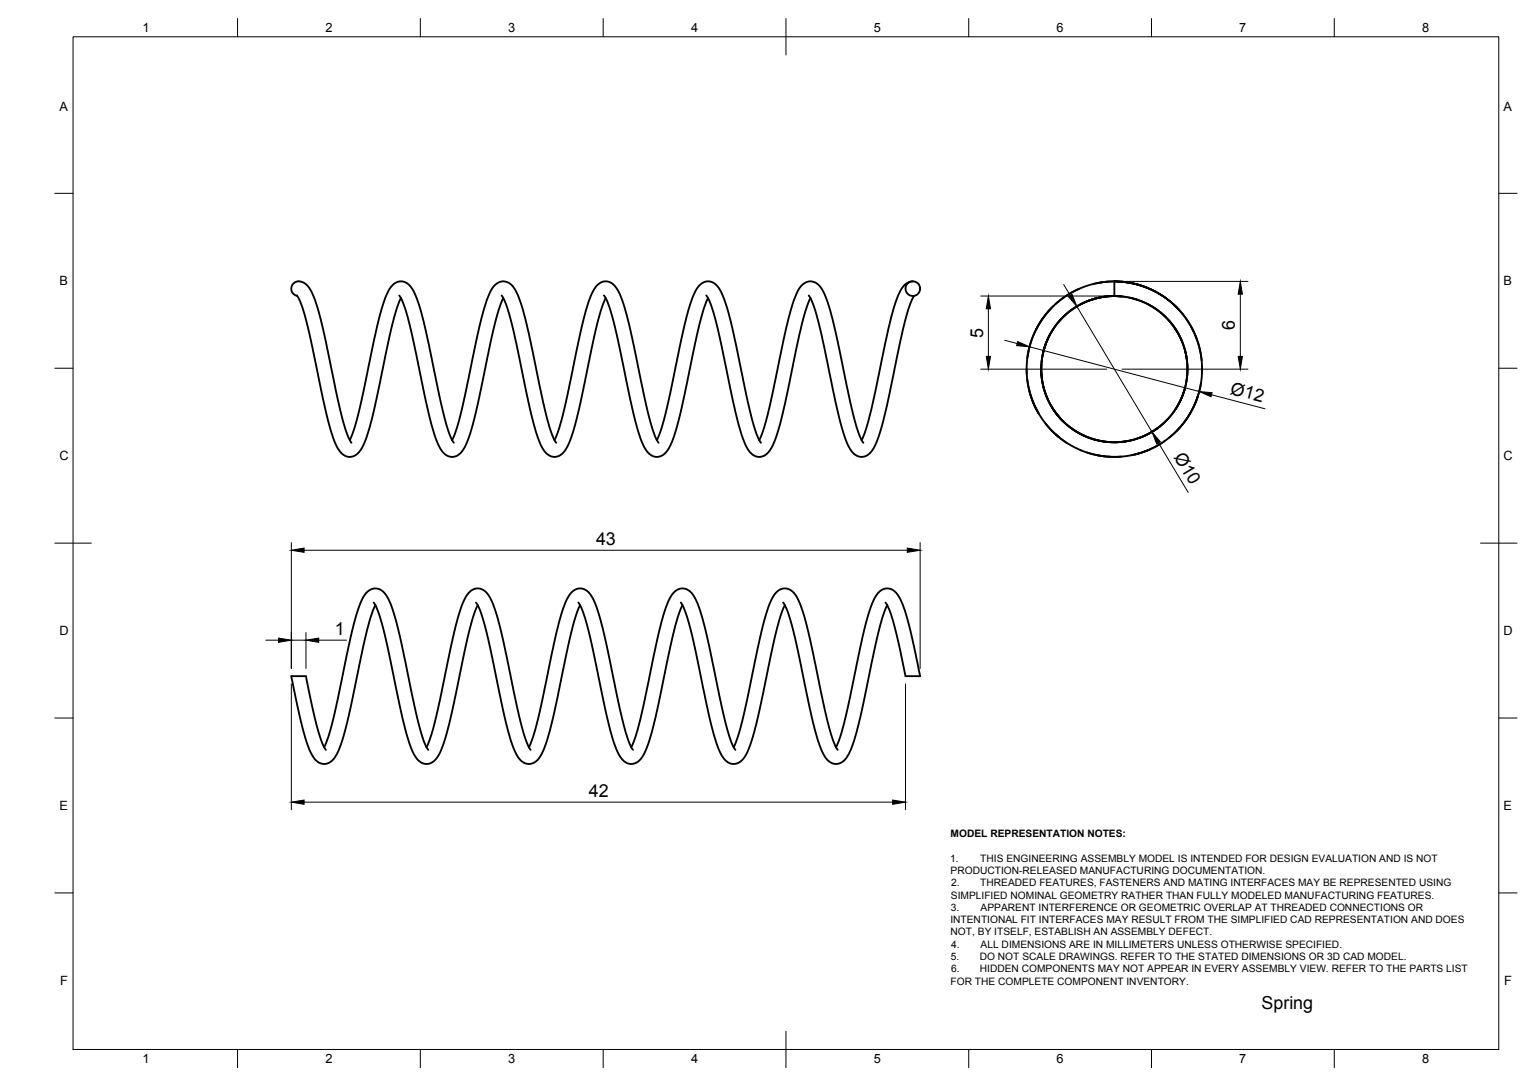
ISO-10303-21;
HEADER;
/* Generated by software containing ST-Developer
 * from STEP Tools, Inc. (www.steptools.com) 
 */

FILE_DESCRIPTION(
/* description */ (''),
/* implementation_level */ '2;1');

FILE_NAME(
/* name */ 'Spring.step',
/* time_stamp */ '2026-10-06T13:05:37-07:00',
/* author */ (''),
/* organization */ (''),
/* preprocessor_version */ 'ST-DEVELOPER v20.2',
/* originating_system */ 'Autodesk Translation Framework v15.15.0.0',
/* authorisation */ '');

FILE_SCHEMA (('AUTOMOTIVE_DESIGN { 1 0 10303 214 3 1 1 }'));
ENDSEC;

DATA;
#10=MECHANICAL_DESIGN_GEOMETRIC_PRESENTATION_REPRESENTATION('',(#145),#28055);
#96=B_SPLINE_SURFACE_WITH_KNOTS('',3,3,((#25876,#25877,#25878,#25879,#25880,
#25881,#25882,#25883,#25884,#25885,#25886,#25887,#25888,#25889,#25890,#25891,
#25892,#25893,#25894,#25895,#25896,#25897,#25898,#25899,#25900,#25901,#25902,
#25903,#25904,#25905,#25906,#25907,#25908,#25909,#25910,#25911,#25912,#25913,
#25914,#25915,#25916,#25917,#25918,#25919,#25920,#25921,#25922,#25923,#25924,
#25925,#25926,#25927,#25928,#25929,#25930,#25931,#25932,#25933,#25934,#25935,
#25936,#25937,#25938,#25939,#25940,#25941,#25942,#25943,#25944,#25945,#25946,
#25947,#25948,#25949,#25950,#25951,#25952,#25953,#25954),(#25955,#25956,
#25957,#25958,#25959,#25960,#25961,#25962,#25963,#25964,#25965,#25966,#25967,
#25968,#25969,#25970,#25971,#25972,#25973,#25974,#25975,#25976,#25977,#25978,
#25979,#25980,#25981,#25982,#25983,#25984,#25985,#25986,#25987,#25988,#25989,
#25990,#25991,#25992,#25993,#25994,#25995,#25996,#25997,#25998,#25999,#26000,
#26001,#26002,#26003,#26004,#26005,#26006,#26007,#26008,#26009,#26010,#26011,
#26012,#26013,#26014,#26015,#26016,#26017,#26018,#26019,#26020,#26021,#26022,
#26023,#26024,#26025,#26026,#26027,#26028,#26029,#26030,#26031,#26032,#26033),
(#26034,#26035,#26036,#26037,#26038,#26039,#26040,#26041,#26042,#26043,
#26044,#26045,#26046,#26047,#26048,#26049,#26050,#26051,#26052,#26053,#26054,
#26055,#26056,#26057,#26058,#26059,#26060,#26061,#26062,#26063,#26064,#26065,
#26066,#26067,#26068,#26069,#26070,#26071,#26072,#26073,#26074,#26075,#26076,
#26077,#26078,#26079,#26080,#26081,#26082,#26083,#26084,#26085,#26086,#26087,
#26088,#26089,#26090,#26091,#26092,#26093,#26094,#26095,#26096,#26097,#26098,
#26099,#26100,#26101,#26102,#26103,#26104,#26105,#26106,#26107,#26108,#26109,
#26110,#26111,#26112),(#26113,#26114,#26115,#26116,#26117,#26118,#26119,
#26120,#26121,#26122,#26123,#26124,#26125,#26126,#26127,#26128,#26129,#26130,
#26131,#26132,#26133,#26134,#26135,#26136,#26137,#26138,#26139,#26140,#26141,
#26142,#26143,#26144,#26145,#26146,#26147,#26148,#26149,#26150,#26151,#26152,
#26153,#26154,#26155,#26156,#26157,#26158,#26159,#26160,#26161,#26162,#26163,
#26164,#26165,#26166,#26167,#26168,#26169,#26170,#26171,#26172,#26173,#26174,
#26175,#26176,#26177,#26178,#26179,#26180,#26181,#26182,#26183,#26184,#26185,
#26186,#26187,#26188,#26189,#26190,#26191),(#26192,#26193,#26194,#26195,
#26196,#26197,#26198,#26199,#26200,#26201,#26202,#26203,#26204,#26205,#26206,
#26207,#26208,#26209,#26210,#26211,#26212,#26213,#26214,#26215,#26216,#26217,
#26218,#26219,#26220,#26221,#26222,#26223,#26224,#26225,#26226,#26227,#26228,
#26229,#26230,#26231,#26232,#26233,#26234,#26235,#26236,#26237,#26238,#26239,
#26240,#26241,#26242,#26243,#26244,#26245,#26246,#26247,#26248,#26249,#26250,
#26251,#26252,#26253,#26254,#26255,#26256,#26257,#26258,#26259,#26260,#26261,
#26262,#26263,#26264,#26265,#26266,#26267,#26268,#26269,#26270),(#26271,
#26272,#26273,#26274,#26275,#26276,#26277,#26278,#26279,#26280,#26281,#26282,
#26283,#26284,#26285,#26286,#26287,#26288,#26289,#26290,#26291,#26292,#26293,
#26294,#26295,#26296,#26297,#26298,#26299,#26300,#26301,#26302,#26303,#26304,
#26305,#26306,#26307,#26308,#26309,#26310,#26311,#26312,#26313,#26314,#26315,
#26316,#26317,#26318,#26319,#26320,#26321,#26322,#26323,#26324,#26325,#26326,
#26327,#26328,#26329,#26330,#26331,#26332,#26333,#26334,#26335,#26336,#26337,
#26338,#26339,#26340,#26341,#26342,#26343,#26344,#26345,#26346,#26347,#26348,
#26349),(#26350,#26351,#26352,#26353,#26354,#26355,#26356,#26357,#26358,
#26359,#26360,#26361,#26362,#26363,#26364,#26365,#26366,#26367,#26368,#26369,
#26370,#26371,#26372,#26373,#26374,#26375,#26376,#26377,#26378,#26379,#26380,
#26381,#26382,#26383,#26384,#26385,#26386,#26387,#26388,#26389,#26390,#26391,
#26392,#26393,#26394,#26395,#26396,#26397,#26398,#26399,#26400,#26401,#26402,
#26403,#26404,#26405,#26406,#26407,#26408,#26409,#26410,#26411,#26412,#26413,
#26414,#26415,#26416,#26417,#26418,#26419,#26420,#26421,#26422,#26423,#26424,
#26425,#26426,#26427,#26428),(#26429,#26430,#26431,#26432,#26433,#26434,
#26435,#26436,#26437,#26438,#26439,#26440,#26441,#26442,#26443,#26444,#26445,
#26446,#26447,#26448,#26449,#26450,#26451,#26452,#26453,#26454,#26455,#26456,
#26457,#26458,#26459,#26460,#26461,#26462,#26463,#26464,#26465,#26466,#26467,
#26468,#26469,#26470,#26471,#26472,#26473,#26474,#26475,#26476,#26477,#26478,
#26479,#26480,#26481,#26482,#26483,#26484,#26485,#26486,#26487,#26488,#26489,
#26490,#26491,#26492,#26493,#26494,#26495,#26496,#26497,#26498,#26499,#26500,
#26501,#26502,#26503,#26504,#26505,#26506,#26507),(#26508,#26509,#26510,
#26511,#26512,#26513,#26514,#26515,#26516,#26517,#26518,#26519,#26520,#26521,
#26522,#26523,#26524,#26525,#26526,#26527,#26528,#26529,#26530,#26531,#26532,
#26533,#26534,#26535,#26536,#26537,#26538,#26539,#26540,#26541,#26542,#26543,
#26544,#26545,#26546,#26547,#26548,#26549,#26550,#26551,#26552,#26553,#26554,
#26555,#26556,#26557,#26558,#26559,#26560,#26561,#26562,#26563,#26564,#26565,
#26566,#26567,#26568,#26569,#26570,#26571,#26572,#26573,#26574,#26575,#26576,
#26577,#26578,#26579,#26580,#26581,#26582,#26583,#26584,#26585,#26586),
(#26587,#26588,#26589,#26590,#26591,#26592,#26593,#26594,#26595,#26596,
#26597,#26598,#26599,#26600,#26601,#26602,#26603,#26604,#26605,#26606,#26607,
#26608,#26609,#26610,#26611,#26612,#26613,#26614,#26615,#26616,#26617,#26618,
#26619,#26620,#26621,#26622,#26623,#26624,#26625,#26626,#26627,#26628,#26629,
#26630,#26631,#26632,#26633,#26634,#26635,#26636,#26637,#26638,#26639,#26640,
#26641,#26642,#26643,#26644,#26645,#26646,#26647,#26648,#26649,#26650,#26651,
#26652,#26653,#26654,#26655,#26656,#26657,#26658,#26659,#26660,#26661,#26662,
#26663,#26664,#26665),(#26666,#26667,#26668,#26669,#26670,#26671,#26672,
#26673,#26674,#26675,#26676,#26677,#26678,#26679,#26680,#26681,#26682,#26683,
#26684,#26685,#26686,#26687,#26688,#26689,#26690,#26691,#26692,#26693,#26694,
#26695,#26696,#26697,#26698,#26699,#26700,#26701,#26702,#26703,#26704,#26705,
#26706,#26707,#26708,#26709,#26710,#26711,#26712,#26713,#26714,#26715,#26716,
#26717,#26718,#26719,#26720,#26721,#26722,#26723,#26724,#26725,#26726,#26727,
#26728,#26729,#26730,#26731,#26732,#26733,#26734,#26735,#26736,#26737,#26738,
#26739,#26740,#26741,#26742,#26743,#26744),(#26745,#26746,#26747,#26748,
#26749,#26750,#26751,#26752,#26753,#26754,#26755,#26756,#26757,#26758,#26759,
#26760,#26761,#26762,#26763,#26764,#26765,#26766,#26767,#26768,#26769,#26770,
#26771,#26772,#26773,#26774,#26775,#26776,#26777,#26778,#26779,#26780,#26781,
#26782,#26783,#26784,#26785,#26786,#26787,#26788,#26789,#26790,#26791,#26792,
#26793,#26794,#26795,#26796,#26797,#26798,#26799,#26800,#26801,#26802,#26803,
#26804,#26805,#26806,#26807,#26808,#26809,#26810,#26811,#26812,#26813,#26814,
#26815,#26816,#26817,#26818,#26819,#26820,#26821,#26822,#26823)),
 .UNSPECIFIED.,.T.,.F.,.F.,(4,1,1,1,2,1,1,1,4),(4,1,1,1,1,1,1,1,1,1,1,1,
1,1,1,1,1,1,1,1,1,1,1,1,1,1,1,1,1,1,1,1,1,1,1,1,1,1,1,1,1,1,1,1,1,1,1,1,
1,1,1,1,1,1,1,1,1,1,1,1,1,1,1,1,1,1,1,1,1,1,1,1,1,1,1,1,4),(-6.28318530717958,
-5.83438635666675,-4.9367884556411,-4.03919055461544,-3.14159265358979,
-2.24399475256414,-1.34639685153848,-0.448798950512828,0.),(0.,0.496040945303652,
0.992081890607303,1.48812283591095,1.98416378121461,2.48020472651826,2.97624567182191,
3.47228661712556,3.96832756242921,4.46436850773286,4.96040945303652,5.45645039834017,
5.95249134364382,6.44853228894747,6.94457323425112,7.44061417955477,7.93665512485842,
8.43269607016208,8.92873701546573,9.42477796076938,9.92081890607303,10.4168598513767,
10.9129007966803,11.408941741984,11.9049826872876,12.4010236325913,12.8970645778949,
13.3931055231986,13.8891464685022,14.3851874138059,14.8812283591095,15.3772693044132,
15.8733102497168,16.3693511950205,16.8653921403242,17.3614330856278,17.8574740309315,
18.3535149762351,18.8495559215388,19.3455968668424,19.8416378121461,20.3376787574497,
20.8337197027534,21.329760648057,21.8258015933607,22.3218425386643,22.817883483968,
23.3139244292716,23.8099653745753,24.3060063198789,24.8020472651826,25.2980882104862,
25.7941291557899,26.2901701010935,26.7862110463972,27.2822519917008,27.7782929370045,
28.2743338823081,28.7703748276118,29.2664157729154,29.7624567182191,30.2584976635227,
30.7545386088264,31.25057955413,31.7466204994337,32.2426614447374,32.738702390041,
33.2347433353447,33.7307842806483,34.226825225952,34.7228661712556,35.2189071165593,
35.7149480618629,36.2109890071666,36.7070299524702,37.2030708977739,37.6991118430775),
 .UNSPECIFIED.);
#97=B_SPLINE_SURFACE_WITH_KNOTS('',3,3,((#27026,#27027,#27028,#27029,#27030,
#27031,#27032,#27033,#27034,#27035,#27036,#27037,#27038,#27039,#27040,#27041,
#27042,#27043,#27044,#27045,#27046,#27047,#27048,#27049,#27050,#27051,#27052,
#27053,#27054,#27055,#27056,#27057,#27058,#27059,#27060,#27061,#27062,#27063,
#27064,#27065,#27066,#27067,#27068,#27069,#27070,#27071,#27072,#27073,#27074,
#27075,#27076,#27077,#27078,#27079,#27080,#27081,#27082,#27083,#27084,#27085,
#27086,#27087,#27088,#27089,#27090,#27091,#27092,#27093,#27094,#27095,#27096,
#27097,#27098,#27099,#27100,#27101,#27102,#27103,#27104),(#27105,#27106,
#27107,#27108,#27109,#27110,#27111,#27112,#27113,#27114,#27115,#27116,#27117,
#27118,#27119,#27120,#27121,#27122,#27123,#27124,#27125,#27126,#27127,#27128,
#27129,#27130,#27131,#27132,#27133,#27134,#27135,#27136,#27137,#27138,#27139,
#27140,#27141,#27142,#27143,#27144,#27145,#27146,#27147,#27148,#27149,#27150,
#27151,#27152,#27153,#27154,#27155,#27156,#27157,#27158,#27159,#27160,#27161,
#27162,#27163,#27164,#27165,#27166,#27167,#27168,#27169,#27170,#27171,#27172,
#27173,#27174,#27175,#27176,#27177,#27178,#27179,#27180,#27181,#27182,#27183),
(#27184,#27185,#27186,#27187,#27188,#27189,#27190,#27191,#27192,#27193,
#27194,#27195,#27196,#27197,#27198,#27199,#27200,#27201,#27202,#27203,#27204,
#27205,#27206,#27207,#27208,#27209,#27210,#27211,#27212,#27213,#27214,#27215,
#27216,#27217,#27218,#27219,#27220,#27221,#27222,#27223,#27224,#27225,#27226,
#27227,#27228,#27229,#27230,#27231,#27232,#27233,#27234,#27235,#27236,#27237,
#27238,#27239,#27240,#27241,#27242,#27243,#27244,#27245,#27246,#27247,#27248,
#27249,#27250,#27251,#27252,#27253,#27254,#27255,#27256,#27257,#27258,#27259,
#27260,#27261,#27262),(#27263,#27264,#27265,#27266,#27267,#27268,#27269,
#27270,#27271,#27272,#27273,#27274,#27275,#27276,#27277,#27278,#27279,#27280,
#27281,#27282,#27283,#27284,#27285,#27286,#27287,#27288,#27289,#27290,#27291,
#27292,#27293,#27294,#27295,#27296,#27297,#27298,#27299,#27300,#27301,#27302,
#27303,#27304,#27305,#27306,#27307,#27308,#27309,#27310,#27311,#27312,#27313,
#27314,#27315,#27316,#27317,#27318,#27319,#27320,#27321,#27322,#27323,#27324,
#27325,#27326,#27327,#27328,#27329,#27330,#27331,#27332,#27333,#27334,#27335,
#27336,#27337,#27338,#27339,#27340,#27341),(#27342,#27343,#27344,#27345,
#27346,#27347,#27348,#27349,#27350,#27351,#27352,#27353,#27354,#27355,#27356,
#27357,#27358,#27359,#27360,#27361,#27362,#27363,#27364,#27365,#27366,#27367,
#27368,#27369,#27370,#27371,#27372,#27373,#27374,#27375,#27376,#27377,#27378,
#27379,#27380,#27381,#27382,#27383,#27384,#27385,#27386,#27387,#27388,#27389,
#27390,#27391,#27392,#27393,#27394,#27395,#27396,#27397,#27398,#27399,#27400,
#27401,#27402,#27403,#27404,#27405,#27406,#27407,#27408,#27409,#27410,#27411,
#27412,#27413,#27414,#27415,#27416,#27417,#27418,#27419,#27420),(#27421,
#27422,#27423,#27424,#27425,#27426,#27427,#27428,#27429,#27430,#27431,#27432,
#27433,#27434,#27435,#27436,#27437,#27438,#27439,#27440,#27441,#27442,#27443,
#27444,#27445,#27446,#27447,#27448,#27449,#27450,#27451,#27452,#27453,#27454,
#27455,#27456,#27457,#27458,#27459,#27460,#27461,#27462,#27463,#27464,#27465,
#27466,#27467,#27468,#27469,#27470,#27471,#27472,#27473,#27474,#27475,#27476,
#27477,#27478,#27479,#27480,#27481,#27482,#27483,#27484,#27485,#27486,#27487,
#27488,#27489,#27490,#27491,#27492,#27493,#27494,#27495,#27496,#27497,#27498,
#27499),(#27500,#27501,#27502,#27503,#27504,#27505,#27506,#27507,#27508,
#27509,#27510,#27511,#27512,#27513,#27514,#27515,#27516,#27517,#27518,#27519,
#27520,#27521,#27522,#27523,#27524,#27525,#27526,#27527,#27528,#27529,#27530,
#27531,#27532,#27533,#27534,#27535,#27536,#27537,#27538,#27539,#27540,#27541,
#27542,#27543,#27544,#27545,#27546,#27547,#27548,#27549,#27550,#27551,#27552,
#27553,#27554,#27555,#27556,#27557,#27558,#27559,#27560,#27561,#27562,#27563,
#27564,#27565,#27566,#27567,#27568,#27569,#27570,#27571,#27572,#27573,#27574,
#27575,#27576,#27577,#27578),(#27579,#27580,#27581,#27582,#27583,#27584,
#27585,#27586,#27587,#27588,#27589,#27590,#27591,#27592,#27593,#27594,#27595,
#27596,#27597,#27598,#27599,#27600,#27601,#27602,#27603,#27604,#27605,#27606,
#27607,#27608,#27609,#27610,#27611,#27612,#27613,#27614,#27615,#27616,#27617,
#27618,#27619,#27620,#27621,#27622,#27623,#27624,#27625,#27626,#27627,#27628,
#27629,#27630,#27631,#27632,#27633,#27634,#27635,#27636,#27637,#27638,#27639,
#27640,#27641,#27642,#27643,#27644,#27645,#27646,#27647,#27648,#27649,#27650,
#27651,#27652,#27653,#27654,#27655,#27656,#27657),(#27658,#27659,#27660,
#27661,#27662,#27663,#27664,#27665,#27666,#27667,#27668,#27669,#27670,#27671,
#27672,#27673,#27674,#27675,#27676,#27677,#27678,#27679,#27680,#27681,#27682,
#27683,#27684,#27685,#27686,#27687,#27688,#27689,#27690,#27691,#27692,#27693,
#27694,#27695,#27696,#27697,#27698,#27699,#27700,#27701,#27702,#27703,#27704,
#27705,#27706,#27707,#27708,#27709,#27710,#27711,#27712,#27713,#27714,#27715,
#27716,#27717,#27718,#27719,#27720,#27721,#27722,#27723,#27724,#27725,#27726,
#27727,#27728,#27729,#27730,#27731,#27732,#27733,#27734,#27735,#27736),
(#27737,#27738,#27739,#27740,#27741,#27742,#27743,#27744,#27745,#27746,
#27747,#27748,#27749,#27750,#27751,#27752,#27753,#27754,#27755,#27756,#27757,
#27758,#27759,#27760,#27761,#27762,#27763,#27764,#27765,#27766,#27767,#27768,
#27769,#27770,#27771,#27772,#27773,#27774,#27775,#27776,#27777,#27778,#27779,
#27780,#27781,#27782,#27783,#27784,#27785,#27786,#27787,#27788,#27789,#27790,
#27791,#27792,#27793,#27794,#27795,#27796,#27797,#27798,#27799,#27800,#27801,
#27802,#27803,#27804,#27805,#27806,#27807,#27808,#27809,#27810,#27811,#27812,
#27813,#27814,#27815),(#27816,#27817,#27818,#27819,#27820,#27821,#27822,
#27823,#27824,#27825,#27826,#27827,#27828,#27829,#27830,#27831,#27832,#27833,
#27834,#27835,#27836,#27837,#27838,#27839,#27840,#27841,#27842,#27843,#27844,
#27845,#27846,#27847,#27848,#27849,#27850,#27851,#27852,#27853,#27854,#27855,
#27856,#27857,#27858,#27859,#27860,#27861,#27862,#27863,#27864,#27865,#27866,
#27867,#27868,#27869,#27870,#27871,#27872,#27873,#27874,#27875,#27876,#27877,
#27878,#27879,#27880,#27881,#27882,#27883,#27884,#27885,#27886,#27887,#27888,
#27889,#27890,#27891,#27892,#27893,#27894),(#27895,#27896,#27897,#27898,
#27899,#27900,#27901,#27902,#27903,#27904,#27905,#27906,#27907,#27908,#27909,
#27910,#27911,#27912,#27913,#27914,#27915,#27916,#27917,#27918,#27919,#27920,
#27921,#27922,#27923,#27924,#27925,#27926,#27927,#27928,#27929,#27930,#27931,
#27932,#27933,#27934,#27935,#27936,#27937,#27938,#27939,#27940,#27941,#27942,
#27943,#27944,#27945,#27946,#27947,#27948,#27949,#27950,#27951,#27952,#27953,
#27954,#27955,#27956,#27957,#27958,#27959,#27960,#27961,#27962,#27963,#27964,
#27965,#27966,#27967,#27968,#27969,#27970,#27971,#27972,#27973)),
 .UNSPECIFIED.,.T.,.F.,.F.,(4,1,1,1,2,1,1,1,4),(4,1,1,1,1,1,1,1,1,1,1,1,
1,1,1,1,1,1,1,1,1,1,1,1,1,1,1,1,1,1,1,1,1,1,1,1,1,1,1,1,1,1,1,1,1,1,1,1,
1,1,1,1,1,1,1,1,1,1,1,1,1,1,1,1,1,1,1,1,1,1,1,1,1,1,1,1,4),(6.28318530717958,
6.73198425769241,7.62958215871806,8.52718005974372,9.42477796076937,10.322375861795,
11.2199737628207,12.1175716638463,12.5663706143592),(0.,0.496040945303652,
0.992081890607303,1.48812283591095,1.98416378121461,2.48020472651826,2.97624567182191,
3.47228661712556,3.96832756242921,4.46436850773286,4.96040945303652,5.45645039834017,
5.95249134364382,6.44853228894747,6.94457323425112,7.44061417955477,7.93665512485842,
8.43269607016208,8.92873701546573,9.42477796076938,9.92081890607303,10.4168598513767,
10.9129007966803,11.408941741984,11.9049826872876,12.4010236325913,12.8970645778949,
13.3931055231986,13.8891464685022,14.3851874138059,14.8812283591095,15.3772693044132,
15.8733102497168,16.3693511950205,16.8653921403242,17.3614330856278,17.8574740309315,
18.3535149762351,18.8495559215388,19.3455968668424,19.8416378121461,20.3376787574497,
20.8337197027534,21.329760648057,21.8258015933607,22.3218425386643,22.817883483968,
23.3139244292716,23.8099653745753,24.3060063198789,24.8020472651826,25.2980882104862,
25.7941291557899,26.2901701010935,26.7862110463972,27.2822519917008,27.7782929370045,
28.2743338823081,28.7703748276118,29.2664157729154,29.7624567182191,30.2584976635227,
30.7545386088264,31.25057955413,31.7466204994337,32.2426614447374,32.738702390041,
33.2347433353447,33.7307842806483,34.226825225952,34.7228661712556,35.2189071165593,
35.7149480618629,36.2109890071666,36.7070299524702,37.2030708977739,37.6991118430775),
 .UNSPECIFIED.);
#125=SHAPE_REPRESENTATION_RELATIONSHIP('SRR','None',#28102,#135);
#135=ADVANCED_BREP_SHAPE_REPRESENTATION('',(#154),#28054);
#145=STYLED_ITEM('',(#28152),#154);
#154=MANIFOLD_SOLID_BREP('Body1',#3688);
#254=PLANE('',#4102);
#255=PLANE('',#4103);
#581=FACE_OUTER_BOUND('',#817,.T.);
#582=FACE_OUTER_BOUND('',#818,.T.);
#583=FACE_OUTER_BOUND('',#819,.T.);
#584=FACE_OUTER_BOUND('',#820,.T.);
#817=EDGE_LOOP('',(#3382,#3383,#3384,#3385));
#818=EDGE_LOOP('',(#3386,#3387,#3388,#3389));
#819=EDGE_LOOP('',(#3390,#3391));
#820=EDGE_LOOP('',(#3392,#3393));
#1388=B_SPLINE_CURVE_WITH_KNOTS('',3,(#26826,#26827,#26828,#26829,#26830,
#26831,#26832,#26833,#26834,#26835,#26836,#26837,#26838,#26839,#26840,#26841,
#26842,#26843,#26844,#26845,#26846,#26847,#26848,#26849,#26850,#26851,#26852,
#26853,#26854,#26855,#26856,#26857,#26858,#26859,#26860,#26861,#26862,#26863,
#26864,#26865,#26866,#26867,#26868,#26869,#26870,#26871,#26872,#26873,#26874,
#26875,#26876,#26877,#26878,#26879,#26880,#26881,#26882,#26883,#26884,#26885,
#26886,#26887,#26888,#26889,#26890,#26891,#26892,#26893,#26894,#26895,#26896,
#26897,#26898,#26899,#26900,#26901,#26902,#26903,#26904),.UNSPECIFIED.,
 .F.,.F.,(4,1,1,1,1,1,1,1,1,1,1,1,1,1,1,1,1,1,1,1,1,1,1,1,1,1,1,1,1,1,1,
1,1,1,1,1,1,1,1,1,1,1,1,1,1,1,1,1,1,1,1,1,1,1,1,1,1,1,1,1,1,1,1,1,1,1,1,
1,1,1,1,1,1,1,1,1,4),(-37.6991118430775,-37.2030708977739,-36.7070299524702,
-36.2109890071666,-35.7149480618629,-35.2189071165593,-34.7228661712556,
-34.226825225952,-33.7307842806483,-33.2347433353447,-32.738702390041,-32.2426614447374,
-31.7466204994337,-31.25057955413,-30.7545386088264,-30.2584976635227,-29.7624567182191,
-29.2664157729154,-28.7703748276118,-28.2743338823081,-27.7782929370045,
-27.2822519917008,-26.7862110463972,-26.2901701010935,-25.7941291557899,
-25.2980882104862,-24.8020472651826,-24.3060063198789,-23.8099653745753,
-23.3139244292716,-22.817883483968,-22.3218425386643,-21.8258015933607,
-21.329760648057,-20.8337197027534,-20.3376787574497,-19.8416378121461,
-19.3455968668424,-18.8495559215388,-18.3535149762351,-17.8574740309315,
-17.3614330856278,-16.8653921403242,-16.3693511950205,-15.8733102497168,
-15.3772693044132,-14.8812283591095,-14.3851874138059,-13.8891464685022,
-13.3931055231986,-12.8970645778949,-12.4010236325913,-11.9049826872876,
-11.408941741984,-10.9129007966803,-10.4168598513767,-9.92081890607303,
-9.42477796076938,-8.92873701546573,-8.43269607016208,-7.93665512485842,
-7.44061417955477,-6.94457323425112,-6.44853228894747,-5.95249134364382,
-5.45645039834017,-4.96040945303652,-4.46436850773286,-3.96832756242921,
-3.47228661712556,-2.97624567182191,-2.48020472651826,-1.98416378121461,
-1.48812283591095,-0.992081890607303,-0.496040945303652,0.),
 .UNSPECIFIED.);
#1389=B_SPLINE_CURVE_WITH_KNOTS('',3,(#26906,#26907,#26908,#26909,#26910,
#26911,#26912,#26913,#26914,#26915,#26916,#26917,#26918,#26919,#26920,#26921,
#26922,#26923,#26924,#26925),.UNSPECIFIED.,.F.,.F.,(4,2,2,2,2,2,2,2,2,4),
(-0.183449247657807,-0.181303576912795,-0.161079000210457,-0.142089796258872,
-0.119840622322675,-0.0936636492746921,-0.0676644266740556,-0.0408453735972391,
-0.019825886307719,-2.33571946147655E-5),.UNSPECIFIED.);
#1390=B_SPLINE_CURVE_WITH_KNOTS('',3,(#26927,#26928,#26929,#26930,#26931,
#26932,#26933,#26934,#26935,#26936,#26937,#26938,#26939,#26940,#26941,#26942,
#26943,#26944,#26945,#26946,#26947,#26948,#26949,#26950,#26951,#26952,#26953,
#26954,#26955,#26956,#26957,#26958,#26959,#26960,#26961,#26962,#26963,#26964,
#26965,#26966,#26967,#26968,#26969,#26970,#26971,#26972,#26973,#26974,#26975,
#26976,#26977,#26978,#26979,#26980,#26981,#26982,#26983,#26984,#26985,#26986,
#26987,#26988,#26989,#26990,#26991,#26992,#26993,#26994,#26995,#26996,#26997,
#26998,#26999,#27000,#27001,#27002,#27003,#27004,#27005),.UNSPECIFIED.,
 .F.,.F.,(4,1,1,1,1,1,1,1,1,1,1,1,1,1,1,1,1,1,1,1,1,1,1,1,1,1,1,1,1,1,1,
1,1,1,1,1,1,1,1,1,1,1,1,1,1,1,1,1,1,1,1,1,1,1,1,1,1,1,1,1,1,1,1,1,1,1,1,
1,1,1,1,1,1,1,1,1,4),(0.,0.496040945303652,0.992081890607303,1.48812283591095,
1.98416378121461,2.48020472651826,2.97624567182191,3.47228661712556,3.96832756242921,
4.46436850773286,4.96040945303652,5.45645039834017,5.95249134364382,6.44853228894747,
6.94457323425112,7.44061417955477,7.93665512485842,8.43269607016208,8.92873701546573,
9.42477796076938,9.92081890607303,10.4168598513767,10.9129007966803,11.408941741984,
11.9049826872876,12.4010236325913,12.8970645778949,13.3931055231986,13.8891464685022,
14.3851874138059,14.8812283591095,15.3772693044132,15.8733102497168,16.3693511950205,
16.8653921403242,17.3614330856278,17.8574740309315,18.3535149762351,18.8495559215388,
19.3455968668424,19.8416378121461,20.3376787574497,20.8337197027534,21.329760648057,
21.8258015933607,22.3218425386643,22.817883483968,23.3139244292716,23.8099653745753,
24.3060063198789,24.8020472651826,25.2980882104862,25.7941291557899,26.2901701010935,
26.7862110463972,27.2822519917008,27.7782929370045,28.2743338823081,28.7703748276118,
29.2664157729154,29.7624567182191,30.2584976635227,30.7545386088264,31.25057955413,
31.7466204994337,32.2426614447374,32.738702390041,33.2347433353447,33.7307842806483,
34.226825225952,34.7228661712556,35.2189071165593,35.7149480618629,36.2109890071666,
36.7070299524702,37.2030708977739,37.6991118430775),.UNSPECIFIED.);
#1391=B_SPLINE_CURVE_WITH_KNOTS('',3,(#27006,#27007,#27008,#27009,#27010,
#27011,#27012,#27013,#27014,#27015,#27016,#27017,#27018,#27019,#27020,#27021,
#27022,#27023,#27024,#27025),.UNSPECIFIED.,.F.,.F.,(4,2,2,2,2,2,2,2,2,4),
(-0.18344924783076,-0.181303577060204,-0.161079000326594,-0.142089796354812,
-0.119840622394364,-0.0936636493252264,-0.067664426704362,-0.0408453736132039,
-0.0198258863122509,-2.33572184239975E-5),.UNSPECIFIED.);
#1392=B_SPLINE_CURVE_WITH_KNOTS('',3,(#27974,#27975,#27976,#27977,#27978,
#27979,#27980,#27981,#27982,#27983,#27984,#27985,#27986,#27987,#27988,#27989,
#27990,#27991,#27992,#27993,#27994,#27995,#27996),.UNSPECIFIED.,.F.,.F.,
(4,3,2,2,2,2,2,2,2,2,4),(-2.33572184239975E-5,0.,0.011884572475286,0.0237029747818905,
0.0434853822238964,0.0621581371447951,0.0836099647869759,0.108563829632263,
0.134733767979787,0.163062104634996,0.182761473566748),.UNSPECIFIED.);
#1393=B_SPLINE_CURVE_WITH_KNOTS('',3,(#27997,#27998,#27999,#28000,#28001,
#28002,#28003,#28004,#28005,#28006,#28007,#28008,#28009,#28010,#28011,#28012,
#28013,#28014,#28015,#28016,#28017,#28018,#28019),.UNSPECIFIED.,.F.,.F.,
(4,3,2,2,2,2,2,2,2,2,4),(-2.33571946147655E-5,0.,0.0118845724779463,0.0237029747888634,
0.0434853822372858,0.0621581371727652,0.0836099648325251,0.108563829705817,
0.134733768045505,0.163062104655266,0.182761473573992),.UNSPECIFIED.);
#1764=VERTEX_POINT('',#26824);
#1765=VERTEX_POINT('',#26825);
#1766=VERTEX_POINT('',#26905);
#1767=VERTEX_POINT('',#26926);
#2304=EDGE_CURVE('',#1764,#1765,#1388,.T.);
#2305=EDGE_CURVE('',#1766,#1764,#1389,.T.);
#2306=EDGE_CURVE('',#1767,#1766,#1390,.T.);
#2307=EDGE_CURVE('',#1767,#1765,#1391,.T.);
#2308=EDGE_CURVE('',#1765,#1767,#1392,.T.);
#2309=EDGE_CURVE('',#1764,#1766,#1393,.T.);
#3382=ORIENTED_EDGE('',*,*,#2304,.F.);
#3383=ORIENTED_EDGE('',*,*,#2305,.F.);
#3384=ORIENTED_EDGE('',*,*,#2306,.F.);
#3385=ORIENTED_EDGE('',*,*,#2307,.T.);
#3386=ORIENTED_EDGE('',*,*,#2304,.T.);
#3387=ORIENTED_EDGE('',*,*,#2308,.T.);
#3388=ORIENTED_EDGE('',*,*,#2306,.T.);
#3389=ORIENTED_EDGE('',*,*,#2309,.F.);
#3390=ORIENTED_EDGE('',*,*,#2305,.T.);
#3391=ORIENTED_EDGE('',*,*,#2309,.T.);
#3392=ORIENTED_EDGE('',*,*,#2307,.F.);
#3393=ORIENTED_EDGE('',*,*,#2308,.F.);
#3673=ADVANCED_FACE('',(#581),#96,.T.);
#3674=ADVANCED_FACE('',(#582),#97,.T.);
#3675=ADVANCED_FACE('',(#583),#254,.T.);
#3676=ADVANCED_FACE('',(#584),#255,.F.);
#3688=CLOSED_SHELL('',(#3673,#3674,#3675,#3676));
#4101=AXIS2_PLACEMENT_3D('',#25875,#4874,#4875);
#4102=AXIS2_PLACEMENT_3D('',#28020,#4876,#4877);
#4103=AXIS2_PLACEMENT_3D('',#28021,#4878,#4879);
#4874=DIRECTION('axis',(0.,0.,1.));
#4875=DIRECTION('refdir',(1.,0.,0.));
#4876=DIRECTION('center_axis',(0.,1.46957615897682E-15,1.));
#4877=DIRECTION('ref_axis',(1.,0.,0.));
#4878=DIRECTION('center_axis',(0.,0.,1.));
#4879=DIRECTION('ref_axis',(1.,0.,0.));
#25875=CARTESIAN_POINT('',(0.,0.,0.));
#25876=CARTESIAN_POINT('Ctrl Pts',(33.9921997677122,5.49976642738082,0.));
#25877=CARTESIAN_POINT('Ctrl Pts',(34.176410294028,5.49976642738082,0.909403588662882));
#25878=CARTESIAN_POINT('Ctrl Pts',(34.5448313466596,5.03991467318512,2.72720954086847));
#25879=CARTESIAN_POINT('Ctrl Pts',(35.0974629256069,3.13419106663809,4.79744756259311));
#25880=CARTESIAN_POINT('Ctrl Pts',(35.6500945045543,0.473252278446431,5.71085179682633));
#25881=CARTESIAN_POINT('Ctrl Pts',(36.2027260835017,-2.30191914515453,5.24783014539696));
#25882=CARTESIAN_POINT('Ctrl Pts',(36.755357662449,-4.52213639346893,3.51971627798693));
#25883=CARTESIAN_POINT('Ctrl Pts',(37.3079892413964,-5.6523152960574,0.943208655172099));
#25884=CARTESIAN_POINT('Ctrl Pts',(37.8606208203438,-5.41997338236277,-1.86068203981508));
#25885=CARTESIAN_POINT('Ctrl Pts',(38.4132523992911,-3.88114100434969,-4.2160410449643));
#25886=CARTESIAN_POINT('Ctrl Pts',(38.9658839782385,-1.40674625429844,-5.55511740772306));
#25887=CARTESIAN_POINT('Ctrl Pts',(39.5185155571859,1.40674646354598,-5.55511666690852));
#25888=CARTESIAN_POINT('Ctrl Pts',(40.0711471361332,3.88114025546219,-4.21604221461142));
#25889=CARTESIAN_POINT('Ctrl Pts',(40.6237787150806,5.41997510425126,-1.86067976428242));
#25890=CARTESIAN_POINT('Ctrl Pts',(41.1764102940279,5.65231160321522,0.943203956408585));
#25891=CARTESIAN_POINT('Ctrl Pts',(41.7290418729754,4.52214418469897,3.51972611893208));
#25892=CARTESIAN_POINT('Ctrl Pts',(42.2816734519227,2.30190265803137,5.24780945677143));
#25893=CARTESIAN_POINT('Ctrl Pts',(42.8343050308701,-0.473218273533045,
5.71089524334113));
#25894=CARTESIAN_POINT('Ctrl Pts',(43.3869366098174,-3.13426874886167,4.79735545609104));
#25895=CARTESIAN_POINT('Ctrl Pts',(43.9395681887648,-5.03979591868312,2.72740116002078));
#25896=CARTESIAN_POINT('Ctrl Pts',(44.4921997677122,-5.73046769283071,-2.96113953592807E-10));
#25897=CARTESIAN_POINT('Ctrl Pts',(45.0448313466595,-5.03979591830015,-2.72740115925713));
#25898=CARTESIAN_POINT('Ctrl Pts',(45.5974629256069,-3.13426874984933,-4.79735545746814));
#25899=CARTESIAN_POINT('Ctrl Pts',(46.1500945045543,-0.473218271369011,
-5.71089524055342));
#25900=CARTESIAN_POINT('Ctrl Pts',(46.7027260835016,2.30190265343826,-5.24780946258346));
#25901=CARTESIAN_POINT('Ctrl Pts',(47.255357662449,4.52214419437993,-3.51972610673135));
#25902=CARTESIAN_POINT('Ctrl Pts',(47.8079892413964,5.65231158284243,-0.943203982060589));
#25903=CARTESIAN_POINT('Ctrl Pts',(48.3606208203438,5.41997514710894,1.86067981823473));
#25904=CARTESIAN_POINT('Ctrl Pts',(48.9132523992911,3.88114016531086,4.21604210112774));
#25905=CARTESIAN_POINT('Ctrl Pts',(49.4658839782385,1.40674665317661,5.55511690561523));
#25906=CARTESIAN_POINT('Ctrl Pts',(50.0185155571858,-1.40674665317677,5.5551169056147));
#25907=CARTESIAN_POINT('Ctrl Pts',(50.5711471361332,-3.8811401653103,4.2160421011286));
#25908=CARTESIAN_POINT('Ctrl Pts',(51.1237787150806,-5.4199751471102,1.86067981823306));
#25909=CARTESIAN_POINT('Ctrl Pts',(51.676410294028,-5.65231158283973,-0.943203982057156));
#25910=CARTESIAN_POINT('Ctrl Pts',(52.2290418729753,-4.52214419438563,-3.51972610673855));
#25911=CARTESIAN_POINT('Ctrl Pts',(52.7816734519227,-2.30190265342625,-5.24780946256834));
#25912=CARTESIAN_POINT('Ctrl Pts',(53.3343050308701,0.473218271343736,-5.71089524058523));
#25913=CARTESIAN_POINT('Ctrl Pts',(53.8869366098175,3.13426874990249,-4.79735545740122));
#25914=CARTESIAN_POINT('Ctrl Pts',(54.4395681887648,5.0397959181883,-2.72740115939791));
#25915=CARTESIAN_POINT('Ctrl Pts',(54.9921997677122,5.73046769306595,-5.11805824213355E-15));
#25916=CARTESIAN_POINT('Ctrl Pts',(55.5448313466596,5.03979591818831,2.72740115939791));
#25917=CARTESIAN_POINT('Ctrl Pts',(56.0974629256069,3.13426874990249,4.79735545740121));
#25918=CARTESIAN_POINT('Ctrl Pts',(56.6500945045543,0.473218271343732,5.71089524058523));
#25919=CARTESIAN_POINT('Ctrl Pts',(57.2027260835016,-2.30190265342626,5.24780946256833));
#25920=CARTESIAN_POINT('Ctrl Pts',(57.755357662449,-4.52214419438564,3.51972610673854));
#25921=CARTESIAN_POINT('Ctrl Pts',(58.3079892413963,-5.65231158283973,0.943203982057152));
#25922=CARTESIAN_POINT('Ctrl Pts',(58.8606208203438,-5.4199751471102,-1.86067981823306));
#25923=CARTESIAN_POINT('Ctrl Pts',(59.4132523992911,-3.88114016531031,-4.2160421011286));
#25924=CARTESIAN_POINT('Ctrl Pts',(59.9658839782385,-1.40674665317677,-5.55511690561469));
#25925=CARTESIAN_POINT('Ctrl Pts',(60.5185155571859,1.40674665317661,-5.55511690561524));
#25926=CARTESIAN_POINT('Ctrl Pts',(61.0711471361332,3.88114016531085,-4.21604210112775));
#25927=CARTESIAN_POINT('Ctrl Pts',(61.6237787150807,5.41997514710894,-1.86067981823474));
#25928=CARTESIAN_POINT('Ctrl Pts',(62.1764102940279,5.65231158284244,0.943203982060585));
#25929=CARTESIAN_POINT('Ctrl Pts',(62.7290418729753,4.52214419437993,3.51972610673135));
#25930=CARTESIAN_POINT('Ctrl Pts',(63.2816734519227,2.30190265343826,5.24780946258346));
#25931=CARTESIAN_POINT('Ctrl Pts',(63.8343050308701,-0.473218271369009,
5.71089524055341));
#25932=CARTESIAN_POINT('Ctrl Pts',(64.3869366098174,-3.13426874984932,4.79735545746814));
#25933=CARTESIAN_POINT('Ctrl Pts',(64.9395681887648,-5.03979591830014,2.72740115925714));
#25934=CARTESIAN_POINT('Ctrl Pts',(65.4921997677122,-5.73046769283071,2.96121409977839E-10));
#25935=CARTESIAN_POINT('Ctrl Pts',(66.0448313466595,-5.03979591868312,-2.72740116002078));
#25936=CARTESIAN_POINT('Ctrl Pts',(66.5974629256069,-3.13426874886167,-4.79735545609105));
#25937=CARTESIAN_POINT('Ctrl Pts',(67.1500945045543,-0.473218273533038,
-5.71089524334112));
#25938=CARTESIAN_POINT('Ctrl Pts',(67.7027260835016,2.30190265803138,-5.24780945677143));
#25939=CARTESIAN_POINT('Ctrl Pts',(68.255357662449,4.52214418469897,-3.51972611893208));
#25940=CARTESIAN_POINT('Ctrl Pts',(68.8079892413964,5.65231160321522,-0.943203956408587));
#25941=CARTESIAN_POINT('Ctrl Pts',(69.3606208203438,5.41997510425126,1.86067976428242));
#25942=CARTESIAN_POINT('Ctrl Pts',(69.9132523992911,3.88114025546219,4.21604221461142));
#25943=CARTESIAN_POINT('Ctrl Pts',(70.4658839782385,1.40674646354597,5.55511666690853));
#25944=CARTESIAN_POINT('Ctrl Pts',(71.0185155571859,-1.40674625429845,5.55511740772306));
#25945=CARTESIAN_POINT('Ctrl Pts',(71.5711471361332,-3.8811410043497,4.21604104496428));
#25946=CARTESIAN_POINT('Ctrl Pts',(72.1237787150806,-5.41997338236277,1.86068203981508));
#25947=CARTESIAN_POINT('Ctrl Pts',(72.676410294028,-5.65231529605741,-0.943208655172103));
#25948=CARTESIAN_POINT('Ctrl Pts',(73.2290418729754,-4.52213639346892,-3.51971627798694));
#25949=CARTESIAN_POINT('Ctrl Pts',(73.7816734519227,-2.30191914515453,-5.24783014539695));
#25950=CARTESIAN_POINT('Ctrl Pts',(74.3343050308701,0.473252278446422,-5.71085179682633));
#25951=CARTESIAN_POINT('Ctrl Pts',(74.8869366098175,3.13419106663809,-4.79744756259312));
#25952=CARTESIAN_POINT('Ctrl Pts',(75.4395681887648,5.03991467318512,-2.72720954086847));
#25953=CARTESIAN_POINT('Ctrl Pts',(75.8079892413964,5.49976642738082,-0.909403588662883));
#25954=CARTESIAN_POINT('Ctrl Pts',(75.9921997677122,5.49976642738082,-8.08232562162E-15));
#25955=CARTESIAN_POINT('Ctrl Pts',(33.9920707665653,5.57474668825,0.));
#25956=CARTESIAN_POINT('Ctrl Pts',(34.1762812928811,5.57474668825,0.921801519276635));
#25957=CARTESIAN_POINT('Ctrl Pts',(34.5447023455127,5.10862550688029,2.76439064201748));
#25958=CARTESIAN_POINT('Ctrl Pts',(35.0973339244601,3.17692056506673,4.86285271511581));
#25959=CARTESIAN_POINT('Ctrl Pts',(35.6499655034074,0.479704279887822,5.78870979651738));
#25960=CARTESIAN_POINT('Ctrl Pts',(36.2025970823548,-2.33330198195422,5.31937556836421));
#25961=CARTESIAN_POINT('Ctrl Pts',(36.7552286613021,-4.5837882052994,3.56770176400508));
#25962=CARTESIAN_POINT('Ctrl Pts',(37.3078602402495,-5.72937521578602,0.956067733435914));
#25963=CARTESIAN_POINT('Ctrl Pts',(37.8604918191969,-5.49386570747434,-1.88604934388851));
#25964=CARTESIAN_POINT('Ctrl Pts',(38.4131233981442,-3.93405390825201,-4.27351975497624));
#25965=CARTESIAN_POINT('Ctrl Pts',(38.9657549770916,-1.42592490042418,-5.63085219620485));
#25966=CARTESIAN_POINT('Ctrl Pts',(39.518386556039,1.42592511248475,-5.63085144582777));
#25967=CARTESIAN_POINT('Ctrl Pts',(40.0710181349864,3.93405314929682,-4.27352093972135));
#25968=CARTESIAN_POINT('Ctrl Pts',(40.6236497139337,5.4938674525111,-1.8860470389829));
#25969=CARTESIAN_POINT('Ctrl Pts',(41.176281292881,5.729371473299,0.95606297402021));
#25970=CARTESIAN_POINT('Ctrl Pts',(41.7289128718285,4.58379610127107,3.56771173198016));
#25971=CARTESIAN_POINT('Ctrl Pts',(42.2815444507758,2.33328527318593,5.31935461269972));
#25972=CARTESIAN_POINT('Ctrl Pts',(42.8341760297232,-0.479669817828385,
5.78875380394745));
#25973=CARTESIAN_POINT('Ctrl Pts',(43.3868076086705,-3.17699929161356,4.8627594207284));
#25974=CARTESIAN_POINT('Ctrl Pts',(43.9394391876179,-5.10850515589866,2.76458473973461));
#25975=CARTESIAN_POINT('Ctrl Pts',(44.4920707665653,-5.80859309124294,-2.99936115018113E-10));
#25976=CARTESIAN_POINT('Ctrl Pts',(45.0447023455126,-5.10850515551054,-2.7645847389611));
#25977=CARTESIAN_POINT('Ctrl Pts',(45.59733392446,-3.17699929261449,-4.86275942212328));
#25978=CARTESIAN_POINT('Ctrl Pts',(46.1499655034074,-0.479669815635259,
-5.78875380112376));
#25979=CARTESIAN_POINT('Ctrl Pts',(46.7025970823548,2.33328526853108,-5.31935461858677));
#25980=CARTESIAN_POINT('Ctrl Pts',(47.2552286613021,4.58379611108217,-3.56771171962194));
#25981=CARTESIAN_POINT('Ctrl Pts',(47.8078602402495,5.72937145265234,-0.956063000003334));
#25982=CARTESIAN_POINT('Ctrl Pts',(48.3604918191969,5.49386749594493,1.88604709363163));
#25983=CARTESIAN_POINT('Ctrl Pts',(48.9131233981442,3.93405305793353,4.27352082477281));
#25984=CARTESIAN_POINT('Ctrl Pts',(49.4657549770916,1.42592530466468,5.63085168761574));
#25985=CARTESIAN_POINT('Ctrl Pts',(50.018386556039,-1.42592530466484,5.6308516876152));
#25986=CARTESIAN_POINT('Ctrl Pts',(50.5710181349864,-3.93405305793297,4.27352082477367));
#25987=CARTESIAN_POINT('Ctrl Pts',(51.1236497139337,-5.49386749594621,1.88604709362994));
#25988=CARTESIAN_POINT('Ctrl Pts',(51.6762812928811,-5.7293714526496,-0.956062999999857));
#25989=CARTESIAN_POINT('Ctrl Pts',(52.2289128718284,-4.58379611108795,-3.56771171962923));
#25990=CARTESIAN_POINT('Ctrl Pts',(52.7815444507759,-2.3332852685189,-5.31935461857145));
#25991=CARTESIAN_POINT('Ctrl Pts',(53.3341760297232,0.479669815609644,-5.78875380115598));
#25992=CARTESIAN_POINT('Ctrl Pts',(53.8868076086706,3.17699929266837,-4.86275942205549));
#25993=CARTESIAN_POINT('Ctrl Pts',(54.4394391876179,5.10850515539719,-2.7645847391037));
#25994=CARTESIAN_POINT('Ctrl Pts',(54.9920707665653,5.80859309148135,-5.41419043299935E-15));
#25995=CARTESIAN_POINT('Ctrl Pts',(55.5447023455127,5.1085051553972,2.7645847391037));
#25996=CARTESIAN_POINT('Ctrl Pts',(56.0973339244601,3.17699929266837,4.86275942205548));
#25997=CARTESIAN_POINT('Ctrl Pts',(56.6499655034074,0.47966981560964,5.78875380115598));
#25998=CARTESIAN_POINT('Ctrl Pts',(57.2025970823548,-2.33328526851891,5.31935461857144));
#25999=CARTESIAN_POINT('Ctrl Pts',(57.7552286613021,-4.58379611108796,3.56771171962922));
#26000=CARTESIAN_POINT('Ctrl Pts',(58.3078602402495,-5.7293714526496,0.956062999999852));
#26001=CARTESIAN_POINT('Ctrl Pts',(58.8604918191969,-5.49386749594621,-1.88604709362995));
#26002=CARTESIAN_POINT('Ctrl Pts',(59.4131233981442,-3.93405305793297,-4.27352082477368));
#26003=CARTESIAN_POINT('Ctrl Pts',(59.9657549770916,-1.42592530466484,-5.63085168761519));
#26004=CARTESIAN_POINT('Ctrl Pts',(60.518386556039,1.42592530466468,-5.63085168761575));
#26005=CARTESIAN_POINT('Ctrl Pts',(61.0710181349863,3.93405305793353,-4.27352082477281));
#26006=CARTESIAN_POINT('Ctrl Pts',(61.6236497139338,5.49386749594494,-1.88604709363164));
#26007=CARTESIAN_POINT('Ctrl Pts',(62.1762812928811,5.72937145265234,0.95606300000333));
#26008=CARTESIAN_POINT('Ctrl Pts',(62.7289128718285,4.58379611108217,3.56771171962194));
#26009=CARTESIAN_POINT('Ctrl Pts',(63.2815444507758,2.33328526853108,5.31935461858677));
#26010=CARTESIAN_POINT('Ctrl Pts',(63.8341760297232,-0.479669815635258,
5.78875380112375));
#26011=CARTESIAN_POINT('Ctrl Pts',(64.3868076086705,-3.17699929261449,4.86275942212328));
#26012=CARTESIAN_POINT('Ctrl Pts',(64.9394391876179,-5.10850515551053,2.76458473896111));
#26013=CARTESIAN_POINT('Ctrl Pts',(65.4920707665653,-5.80859309124295,2.9994369153224E-10));
#26014=CARTESIAN_POINT('Ctrl Pts',(66.0447023455127,-5.10850515589866,-2.76458473973461));
#26015=CARTESIAN_POINT('Ctrl Pts',(66.59733392446,-3.17699929161356,-4.86275942072841));
#26016=CARTESIAN_POINT('Ctrl Pts',(67.1499655034074,-0.479669817828379,
-5.78875380394745));
#26017=CARTESIAN_POINT('Ctrl Pts',(67.7025970823548,2.33328527318594,-5.31935461269972));
#26018=CARTESIAN_POINT('Ctrl Pts',(68.2552286613022,4.58379610127107,-3.56771173198016));
#26019=CARTESIAN_POINT('Ctrl Pts',(68.8078602402495,5.72937147329901,-0.956062974020212));
#26020=CARTESIAN_POINT('Ctrl Pts',(69.3604918191969,5.4938674525111,1.8860470389829));
#26021=CARTESIAN_POINT('Ctrl Pts',(69.9131233981443,3.93405314929682,4.27352093972134));
#26022=CARTESIAN_POINT('Ctrl Pts',(70.4657549770917,1.42592511248473,5.63085144582777));
#26023=CARTESIAN_POINT('Ctrl Pts',(71.018386556039,-1.42592490042419,5.63085219620485));
#26024=CARTESIAN_POINT('Ctrl Pts',(71.5710181349864,-3.93405390825202,4.27351975497623));
#26025=CARTESIAN_POINT('Ctrl Pts',(72.1236497139337,-5.49386570747434,1.88604934388851));
#26026=CARTESIAN_POINT('Ctrl Pts',(72.6762812928811,-5.72937521578603,-0.956067733435918));
#26027=CARTESIAN_POINT('Ctrl Pts',(73.2289128718285,-4.58378820529939,-3.56770176400509));
#26028=CARTESIAN_POINT('Ctrl Pts',(73.7815444507758,-2.33330198195422,-5.31937556836421));
#26029=CARTESIAN_POINT('Ctrl Pts',(74.3341760297232,0.479704279887813,-5.78870979651738));
#26030=CARTESIAN_POINT('Ctrl Pts',(74.8868076086706,3.17692056506672,-4.86285271511582));
#26031=CARTESIAN_POINT('Ctrl Pts',(75.4394391876179,5.10862550688029,-2.76439064201748));
#26032=CARTESIAN_POINT('Ctrl Pts',(75.8078602402495,5.57474668825,-0.921801519276636));
#26033=CARTESIAN_POINT('Ctrl Pts',(75.9920707665653,5.57474668825,-8.19251482538721E-15));
#26034=CARTESIAN_POINT('Ctrl Pts',(33.9431414536155,5.79981109503712,0.));
#26035=CARTESIAN_POINT('Ctrl Pts',(34.1273519799313,5.79981109503712,0.95899747143683));
#26036=CARTESIAN_POINT('Ctrl Pts',(34.4957730325629,5.31486464408031,2.87600085013837));
#26037=CARTESIAN_POINT('Ctrl Pts',(35.0484046115103,3.30517718677737,5.05916675657821));
#26038=CARTESIAN_POINT('Ctrl Pts',(35.6010361904576,0.499070024096898,6.02240821551781));
#26039=CARTESIAN_POINT('Ctrl Pts',(36.153667769405,-2.42749964852484,5.53412340547436));
#26040=CARTESIAN_POINT('Ctrl Pts',(36.7062993483523,-4.76884068918239,3.71173413415615));
#26041=CARTESIAN_POINT('Ctrl Pts',(37.2589309272997,-5.96067611682369,0.994664977192594));
#26042=CARTESIAN_POINT('Ctrl Pts',(37.8115625062471,-5.71565890873659,-1.96219104782992));
#26043=CARTESIAN_POINT('Ctrl Pts',(38.3641940851944,-4.09287582201278,-4.4460463256512));
#26044=CARTESIAN_POINT('Ctrl Pts',(38.9168256641418,-1.48349100436533,-5.85817564103365));
#26045=CARTESIAN_POINT('Ctrl Pts',(39.4694572430892,1.48349122236704,-5.85817489580175));
#26046=CARTESIAN_POINT('Ctrl Pts',(40.0220888220366,4.09287504179451,-4.44604750227257));
#26047=CARTESIAN_POINT('Ctrl Pts',(40.5747204009839,5.71566070266274,-1.96218875872725));
#26048=CARTESIAN_POINT('Ctrl Pts',(41.1273519799312,5.96067226948622,0.994660250423079));
#26049=CARTESIAN_POINT('Ctrl Pts',(41.6799835588787,4.76884880636957,3.71174403388056));
#26050=CARTESIAN_POINT('Ctrl Pts',(42.232615137826,2.42748247163953,5.5341025943587));
#26051=CARTESIAN_POINT('Ctrl Pts',(42.7852467167734,-0.499034596539813,
6.0224519278597));
#26052=CARTESIAN_POINT('Ctrl Pts',(43.3378782957207,-3.30525811894677,5.0590741705265));
#26053=CARTESIAN_POINT('Ctrl Pts',(43.8905098746681,-5.31474092131558,2.87619395462708));
#26054=CARTESIAN_POINT('Ctrl Pts',(44.4431414536155,-6.04309214833711,-2.97879057897562E-10));
#26055=CARTESIAN_POINT('Ctrl Pts',(44.9957730325628,-5.31474092091659,-2.87619395385888));
#26056=CARTESIAN_POINT('Ctrl Pts',(45.5484046115102,-3.30525811997574,-5.05907417191182));
#26057=CARTESIAN_POINT('Ctrl Pts',(46.1010361904576,-0.499034594285245,
-6.02245192505537));
#26058=CARTESIAN_POINT('Ctrl Pts',(46.653667769405,2.42748246685427,-5.53410260020539));
#26059=CARTESIAN_POINT('Ctrl Pts',(47.2062993483523,4.76884881645555,-3.71174402160707));
#26060=CARTESIAN_POINT('Ctrl Pts',(47.7589309272997,5.96067224826112,-0.994660276228043));
#26061=CARTESIAN_POINT('Ctrl Pts',(48.3115625062471,5.71566074731342,1.96218881300126));
#26062=CARTESIAN_POINT('Ctrl Pts',(48.8641940851944,4.09287494787157,4.44604738811221));
#26063=CARTESIAN_POINT('Ctrl Pts',(49.4168256641418,1.48349141993114,5.85817513593182));
#26064=CARTESIAN_POINT('Ctrl Pts',(49.9694572430891,-1.48349141993129,5.85817513593129));
#26065=CARTESIAN_POINT('Ctrl Pts',(50.5220888220366,-4.09287494787099,4.44604738811307));
#26066=CARTESIAN_POINT('Ctrl Pts',(51.0747204009839,-5.71566074731474,1.96218881299959));
#26067=CARTESIAN_POINT('Ctrl Pts',(51.6273519799313,-5.96067224825831,-0.994660276224589));
#26068=CARTESIAN_POINT('Ctrl Pts',(52.1799835588786,-4.76884881646149,-3.71174402161432));
#26069=CARTESIAN_POINT('Ctrl Pts',(52.7326151378261,-2.42748246684175,-5.53410260019018));
#26070=CARTESIAN_POINT('Ctrl Pts',(53.2852467167734,0.499034594258913,-6.02245192508737));
#26071=CARTESIAN_POINT('Ctrl Pts',(53.8378782957208,3.30525812003113,-5.0590741718445));
#26072=CARTESIAN_POINT('Ctrl Pts',(54.3905098746681,5.31474092080006,-2.8761939540005));
#26073=CARTESIAN_POINT('Ctrl Pts',(54.9431414536155,6.0430921485822,-6.36963580352865E-15));
#26074=CARTESIAN_POINT('Ctrl Pts',(55.4957730325629,5.31474092080007,2.8761939540005));
#26075=CARTESIAN_POINT('Ctrl Pts',(56.0484046115103,3.30525812003113,5.05907417184449));
#26076=CARTESIAN_POINT('Ctrl Pts',(56.6010361904576,0.499034594258907,6.02245192508737));
#26077=CARTESIAN_POINT('Ctrl Pts',(57.1536677694049,-2.42748246684176,5.53410260019017));
#26078=CARTESIAN_POINT('Ctrl Pts',(57.7062993483523,-4.7688488164615,3.71174402161431));
#26079=CARTESIAN_POINT('Ctrl Pts',(58.2589309272996,-5.9606722482583,0.994660276224585));
#26080=CARTESIAN_POINT('Ctrl Pts',(58.8115625062471,-5.71566074731474,-1.96218881299959));
#26081=CARTESIAN_POINT('Ctrl Pts',(59.3641940851944,-4.09287494787099,-4.44604738811308));
#26082=CARTESIAN_POINT('Ctrl Pts',(59.9168256641418,-1.4834914199313,-5.85817513593128));
#26083=CARTESIAN_POINT('Ctrl Pts',(60.4694572430892,1.48349141993113,-5.85817513593183));
#26084=CARTESIAN_POINT('Ctrl Pts',(61.0220888220365,4.09287494787156,-4.44604738811222));
#26085=CARTESIAN_POINT('Ctrl Pts',(61.574720400984,5.71566074731343,-1.96218881300128));
#26086=CARTESIAN_POINT('Ctrl Pts',(62.1273519799312,5.96067224826113,0.994660276228038));
#26087=CARTESIAN_POINT('Ctrl Pts',(62.6799835588787,4.76884881645555,3.71174402160707));
#26088=CARTESIAN_POINT('Ctrl Pts',(63.232615137826,2.42748246685427,5.53410260020538));
#26089=CARTESIAN_POINT('Ctrl Pts',(63.7852467167734,-0.499034594285243,
6.02245192505537));
#26090=CARTESIAN_POINT('Ctrl Pts',(64.3378782957207,-3.30525811997573,5.05907417191182));
#26091=CARTESIAN_POINT('Ctrl Pts',(64.8905098746681,-5.31474092091658,2.87619395385889));
#26092=CARTESIAN_POINT('Ctrl Pts',(65.4431414536155,-6.04309214833712,2.97887036704478E-10));
#26093=CARTESIAN_POINT('Ctrl Pts',(65.9957730325628,-5.31474092131558,-2.87619395462708));
#26094=CARTESIAN_POINT('Ctrl Pts',(66.5484046115102,-3.30525811894677,-5.05907417052651));
#26095=CARTESIAN_POINT('Ctrl Pts',(67.1010361904576,-0.499034596539806,
-6.0224519278597));
#26096=CARTESIAN_POINT('Ctrl Pts',(67.653667769405,2.42748247163954,-5.5341025943587));
#26097=CARTESIAN_POINT('Ctrl Pts',(68.2062993483523,4.76884880636957,-3.71174403388056));
#26098=CARTESIAN_POINT('Ctrl Pts',(68.7589309272997,5.96067226948623,-0.994660250423083));
#26099=CARTESIAN_POINT('Ctrl Pts',(69.3115625062471,5.71566070266274,1.96218875872725));
#26100=CARTESIAN_POINT('Ctrl Pts',(69.8641940851944,4.09287504179451,4.44604750227256));
#26101=CARTESIAN_POINT('Ctrl Pts',(70.4168256641419,1.48349122236702,5.85817489580176));
#26102=CARTESIAN_POINT('Ctrl Pts',(70.9694572430892,-1.48349100436534,5.85817564103365));
#26103=CARTESIAN_POINT('Ctrl Pts',(71.5220888220366,-4.09287582201279,4.44604632565119));
#26104=CARTESIAN_POINT('Ctrl Pts',(72.0747204009839,-5.71565890873659,1.96219104782992));
#26105=CARTESIAN_POINT('Ctrl Pts',(72.6273519799313,-5.9606761168237,-0.994664977192599));
#26106=CARTESIAN_POINT('Ctrl Pts',(73.1799835588787,-4.76884068918239,-3.71173413415616));
#26107=CARTESIAN_POINT('Ctrl Pts',(73.732615137826,-2.42749964852484,-5.53412340547436));
#26108=CARTESIAN_POINT('Ctrl Pts',(74.2852467167734,0.499070024096889,-6.02240821551781));
#26109=CARTESIAN_POINT('Ctrl Pts',(74.8378782957208,3.30517718677736,-5.05916675657822));
#26110=CARTESIAN_POINT('Ctrl Pts',(75.3905098746681,5.31486464408031,-2.87600085013837));
#26111=CARTESIAN_POINT('Ctrl Pts',(75.7589309272997,5.79981109503712,-0.958997471436831));
#26112=CARTESIAN_POINT('Ctrl Pts',(75.9431414536155,5.79981109503712,-8.52326411183583E-15));
#26113=CARTESIAN_POINT('Ctrl Pts',(33.62030855087,6.05892730518855,0.));
#26114=CARTESIAN_POINT('Ctrl Pts',(33.8045190771858,6.05892730518855,1.00170122537842));
#26115=CARTESIAN_POINT('Ctrl Pts',(34.1729401298174,5.55226374371841,3.00453419845087));
#26116=CARTESIAN_POINT('Ctrl Pts',(34.7255717087647,3.45282354398353,5.28512205116659));
#26117=CARTESIAN_POINT('Ctrl Pts',(35.2782032877121,0.52135987967838,6.29143885263431));
#26118=CARTESIAN_POINT('Ctrl Pts',(35.8308348666595,-2.53593227701648,5.78132024999939));
#26119=CARTESIAN_POINT('Ctrl Pts',(36.3834664456069,-4.98186108464976,3.87753730806675));
#26120=CARTESIAN_POINT('Ctrl Pts',(36.9360980245542,-6.22693362925883,1.03909408852531));
#26121=CARTESIAN_POINT('Ctrl Pts',(37.4887296035016,-5.97097223597331,-2.04983951271052));
#26122=CARTESIAN_POINT('Ctrl Pts',(38.0413611824489,-4.27570069868504,-4.64464744982032));
#26123=CARTESIAN_POINT('Ctrl Pts',(38.5939927613963,-1.54975720378295,-6.11985471822127));
#26124=CARTESIAN_POINT('Ctrl Pts',(39.1466243403437,1.54975741221459,-6.11985420086809));
#26125=CARTESIAN_POINT('Ctrl Pts',(39.6992559192911,4.27569995271762,-4.64464826665024));
#26126=CARTESIAN_POINT('Ctrl Pts',(40.2518874982384,5.97097395114776,-2.04983792356467));
#26127=CARTESIAN_POINT('Ctrl Pts',(40.8045190771858,6.22692995081589,1.03909080720973));
#26128=CARTESIAN_POINT('Ctrl Pts',(41.3571506561332,4.98186884549998,3.87754418138483));
#26129=CARTESIAN_POINT('Ctrl Pts',(41.9097822350805,2.53591585418045,5.78130580919469));
#26130=CARTESIAN_POINT('Ctrl Pts',(42.4624138140279,-0.521326007358065,
6.29146924994462));
#26131=CARTESIAN_POINT('Ctrl Pts',(43.0150453929753,-3.45290092330605,5.28505830615491));
#26132=CARTESIAN_POINT('Ctrl Pts',(43.5676769719227,-5.55214545226785,3.00467086174248));
#26133=CARTESIAN_POINT('Ctrl Pts',(44.12030855087,-6.31303145085601,-2.06792707167108E-10));
#26134=CARTESIAN_POINT('Ctrl Pts',(44.6729401298174,-5.55214545188636,-3.00467086120918));
#26135=CARTESIAN_POINT('Ctrl Pts',(45.2255717087647,-3.45290092428985,-5.28505830711662));
#26136=CARTESIAN_POINT('Ctrl Pts',(45.7782032877121,-0.521326005202469,
-6.29146924799781));
#26137=CARTESIAN_POINT('Ctrl Pts',(46.3308348666595,2.53591584960525,-5.78130581325357));
#26138=CARTESIAN_POINT('Ctrl Pts',(46.8834664456069,4.98186885514319,-3.87754417286436));
#26139=CARTESIAN_POINT('Ctrl Pts',(47.4360980245542,6.22692993052255,-1.03909082512399));
#26140=CARTESIAN_POINT('Ctrl Pts',(47.9887296035015,5.97097399383832,2.04983796124264));
#26141=CARTESIAN_POINT('Ctrl Pts',(48.541361182449,4.27569986291781,4.64464818739812));
#26142=CARTESIAN_POINT('Ctrl Pts',(49.0939927613963,1.54975760110581,6.11985436757058));
#26143=CARTESIAN_POINT('Ctrl Pts',(49.6466243403437,-1.54975760110596,6.11985436757021));
#26144=CARTESIAN_POINT('Ctrl Pts',(50.199255919291,-4.27569986291726,4.64464818739871));
#26145=CARTESIAN_POINT('Ctrl Pts',(50.7518874982385,-5.97097399383958,2.04983796124148));
#26146=CARTESIAN_POINT('Ctrl Pts',(51.3045190771858,-6.22692993051986,-1.03909082512159));
#26147=CARTESIAN_POINT('Ctrl Pts',(51.8571506561332,-4.98186885514887,-3.87754417286939));
#26148=CARTESIAN_POINT('Ctrl Pts',(52.4097822350806,-2.53591584959328,-5.781305813243));
#26149=CARTESIAN_POINT('Ctrl Pts',(52.9624138140279,0.521326005177292,-6.29146924802002));
#26150=CARTESIAN_POINT('Ctrl Pts',(53.5150453929753,3.45290092434281,-5.28505830706988));
#26151=CARTESIAN_POINT('Ctrl Pts',(54.0676769719227,5.55214545177497,-3.0046708613075));
#26152=CARTESIAN_POINT('Ctrl Pts',(54.62030855087,6.31303145109033,-5.36390383455044E-15));
#26153=CARTESIAN_POINT('Ctrl Pts',(55.1729401298174,5.55214545177497,3.0046708613075));
#26154=CARTESIAN_POINT('Ctrl Pts',(55.7255717087647,3.45290092434281,5.28505830706987));
#26155=CARTESIAN_POINT('Ctrl Pts',(56.2782032877121,0.521326005177289,6.29146924802003));
#26156=CARTESIAN_POINT('Ctrl Pts',(56.8308348666595,-2.5359158495933,5.781305813243));
#26157=CARTESIAN_POINT('Ctrl Pts',(57.3834664456068,-4.98186885514888,3.87754417286939));
#26158=CARTESIAN_POINT('Ctrl Pts',(57.9360980245542,-6.22692993051986,1.03909082512159));
#26159=CARTESIAN_POINT('Ctrl Pts',(58.4887296035016,-5.97097399383958,-2.04983796124148));
#26160=CARTESIAN_POINT('Ctrl Pts',(59.041361182449,-4.27569986291726,-4.64464818739871));
#26161=CARTESIAN_POINT('Ctrl Pts',(59.5939927613963,-1.54975760110596,-6.11985436757021));
#26162=CARTESIAN_POINT('Ctrl Pts',(60.1466243403437,1.5497576011058,-6.11985436757059));
#26163=CARTESIAN_POINT('Ctrl Pts',(60.699255919291,4.2756998629178,-4.64464818739812));
#26164=CARTESIAN_POINT('Ctrl Pts',(61.2518874982385,5.97097399383833,-2.04983796124265));
#26165=CARTESIAN_POINT('Ctrl Pts',(61.8045190771858,6.22692993052255,1.03909082512398));
#26166=CARTESIAN_POINT('Ctrl Pts',(62.3571506561332,4.98186885514319,3.87754417286436));
#26167=CARTESIAN_POINT('Ctrl Pts',(62.9097822350805,2.53591584960525,5.78130581325356));
#26168=CARTESIAN_POINT('Ctrl Pts',(63.4624138140279,-0.521326005202466,
6.2914692479978));
#26169=CARTESIAN_POINT('Ctrl Pts',(64.0150453929752,-3.45290092428985,5.28505830711661));
#26170=CARTESIAN_POINT('Ctrl Pts',(64.5676769719227,-5.55214545188636,3.00467086120919));
#26171=CARTESIAN_POINT('Ctrl Pts',(65.1203085508701,-6.31303145085602,2.06801021218025E-10));
#26172=CARTESIAN_POINT('Ctrl Pts',(65.6729401298174,-5.55214545226785,-3.00467086174248));
#26173=CARTESIAN_POINT('Ctrl Pts',(66.2255717087647,-3.45290092330605,-5.28505830615491));
#26174=CARTESIAN_POINT('Ctrl Pts',(66.7782032877121,-0.521326007358057,
-6.29146924994462));
#26175=CARTESIAN_POINT('Ctrl Pts',(67.3308348666595,2.53591585418046,-5.78130580919469));
#26176=CARTESIAN_POINT('Ctrl Pts',(67.8834664456069,4.98186884549998,-3.87754418138483));
#26177=CARTESIAN_POINT('Ctrl Pts',(68.4360980245542,6.22692995081589,-1.03909080720973));
#26178=CARTESIAN_POINT('Ctrl Pts',(68.9887296035016,5.97097395114776,2.04983792356467));
#26179=CARTESIAN_POINT('Ctrl Pts',(69.541361182449,4.27569995271762,4.64464826665024));
#26180=CARTESIAN_POINT('Ctrl Pts',(70.0939927613963,1.54975741221458,6.1198542008681));
#26181=CARTESIAN_POINT('Ctrl Pts',(70.6466243403438,-1.54975720378297,6.11985471822127));
#26182=CARTESIAN_POINT('Ctrl Pts',(71.199255919291,-4.27570069868505,4.6446474498203));
#26183=CARTESIAN_POINT('Ctrl Pts',(71.7518874982385,-5.9709722359733,2.04983951271053));
#26184=CARTESIAN_POINT('Ctrl Pts',(72.3045190771858,-6.22693362925883,-1.03909408852532));
#26185=CARTESIAN_POINT('Ctrl Pts',(72.8571506561333,-4.98186108464976,-3.87753730806676));
#26186=CARTESIAN_POINT('Ctrl Pts',(73.4097822350805,-2.53593227701648,-5.78132024999937));
#26187=CARTESIAN_POINT('Ctrl Pts',(73.962413814028,0.521359879678368,-6.29143885263431));
#26188=CARTESIAN_POINT('Ctrl Pts',(74.5150453929753,3.45282354398353,-5.2851220511666));
#26189=CARTESIAN_POINT('Ctrl Pts',(75.0676769719227,5.55226374371841,-3.00453419845087));
#26190=CARTESIAN_POINT('Ctrl Pts',(75.4360980245542,6.05892730518855,-1.00170122537842));
#26191=CARTESIAN_POINT('Ctrl Pts',(75.62030855087,6.05892730518855,-8.90405511667878E-15));
#26192=CARTESIAN_POINT('Ctrl Pts',(33.1358237202237,5.94680344913766,0.));
#26193=CARTESIAN_POINT('Ctrl Pts',(33.3200342465395,5.94680344913766,0.983379197578396));
#26194=CARTESIAN_POINT('Ctrl Pts',(33.6884552991711,5.44959421336945,2.94886771297254));
#26195=CARTESIAN_POINT('Ctrl Pts',(34.2410868781184,3.38895443893944,5.18742673184628));
#26196=CARTESIAN_POINT('Ctrl Pts',(34.7937184570658,0.511722382884761,6.17505868653612));
#26197=CARTESIAN_POINT('Ctrl Pts',(35.3463500360132,-2.48903384632581,5.67440885923965));
#26198=CARTESIAN_POINT('Ctrl Pts',(35.8989816149605,-4.88972305399822,3.80581898848347));
#26199=CARTESIAN_POINT('Ctrl Pts',(36.4516131939079,-6.11177024810298,1.01987909450271));
#26200=CARTESIAN_POINT('Ctrl Pts',(37.0042447728553,-5.86054195732468,-2.01192998939814));
#26201=CARTESIAN_POINT('Ctrl Pts',(37.5568763518026,-4.19662395290879,-4.55874653989111));
#26202=CARTESIAN_POINT('Ctrl Pts',(38.10950793075,-1.52109519307483,-6.00667145344936));
#26203=CARTESIAN_POINT('Ctrl Pts',(38.6621395096974,1.5210954270842,-6.00667054754812));
#26204=CARTESIAN_POINT('Ctrl Pts',(39.2147710886447,4.19662311539983,-4.55874797018865));
#26205=CARTESIAN_POINT('Ctrl Pts',(39.7674026675921,5.86054388297712,-2.01192720677863));
#26206=CARTESIAN_POINT('Ctrl Pts',(40.3200342465395,6.11176611825916,1.01987334860882));
#26207=CARTESIAN_POINT('Ctrl Pts',(40.8726658254868,4.88973176722276,3.80583102214387));
#26208=CARTESIAN_POINT('Ctrl Pts',(41.4252974044342,2.4890154081581,5.67438355771667));
#26209=CARTESIAN_POINT('Ctrl Pts',(41.9779289833816,-0.511684353915735,
6.17511179518466));
#26210=CARTESIAN_POINT('Ctrl Pts',(42.5305605623289,-3.38904131388133,5.18731389692575));
#26211=CARTESIAN_POINT('Ctrl Pts',(43.0831921412763,-5.44946140575937,2.9491010349948));
#26212=CARTESIAN_POINT('Ctrl Pts',(43.6358237202237,-6.19627521287463,-3.62104274501345E-10));
#26213=CARTESIAN_POINT('Ctrl Pts',(44.1884552991711,-5.44946140533107,-2.94910103406097));
#26214=CARTESIAN_POINT('Ctrl Pts',(44.7410868781184,-3.38904131498586,-5.18731389860973));
#26215=CARTESIAN_POINT('Ctrl Pts',(45.2937184570658,-0.511684351495615,
-6.17511179177572));
#26216=CARTESIAN_POINT('Ctrl Pts',(45.8463500360132,2.48901540302145,-5.67438356482389));
#26217=CARTESIAN_POINT('Ctrl Pts',(46.3989816149605,4.88973177804935,-3.80583100722426));
#26218=CARTESIAN_POINT('Ctrl Pts',(46.9516131939079,6.11176609547551,-1.01987337997725));
#26219=CARTESIAN_POINT('Ctrl Pts',(47.5042447728553,5.86054393090647,2.01192727275394));
#26220=CARTESIAN_POINT('Ctrl Pts',(48.0568763518026,4.19662301458021,4.55874783141572));
#26221=CARTESIAN_POINT('Ctrl Pts',(48.60950793075,1.52109563915525,6.00667083944942));
#26222=CARTESIAN_POINT('Ctrl Pts',(49.1621395096974,-1.52109563915541,6.00667083944875));
#26223=CARTESIAN_POINT('Ctrl Pts',(49.7147710886447,-4.1966230145796,4.55874783141676));
#26224=CARTESIAN_POINT('Ctrl Pts',(50.2674026675921,-5.86054393090788,2.0119272727519));
#26225=CARTESIAN_POINT('Ctrl Pts',(50.8200342465394,-6.1117660954725,-1.01987337997305));
#26226=CARTESIAN_POINT('Ctrl Pts',(51.3726658254868,-4.88973177805572,-3.80583100723307));
#26227=CARTESIAN_POINT('Ctrl Pts',(51.9252974044342,-2.48901540300802,-5.67438356480538));
#26228=CARTESIAN_POINT('Ctrl Pts',(52.4779289833816,0.511684351467352,-6.17511179181463));
#26229=CARTESIAN_POINT('Ctrl Pts',(53.030560562329,3.38904131504531,-5.18731389852789));
#26230=CARTESIAN_POINT('Ctrl Pts',(53.5831921412763,5.449461405206,-2.94910103423313));
#26231=CARTESIAN_POINT('Ctrl Pts',(54.1358237202237,6.1962752131377,-6.168489409733E-15));
#26232=CARTESIAN_POINT('Ctrl Pts',(54.688455299171,5.44946140520601,2.94910103423312));
#26233=CARTESIAN_POINT('Ctrl Pts',(55.2410868781184,3.38904131504531,5.18731389852788));
#26234=CARTESIAN_POINT('Ctrl Pts',(55.7937184570658,0.511684351467345,6.17511179181463));
#26235=CARTESIAN_POINT('Ctrl Pts',(56.3463500360131,-2.48901540300803,5.67438356480538));
#26236=CARTESIAN_POINT('Ctrl Pts',(56.8989816149606,-4.88973177805573,3.80583100723306));
#26237=CARTESIAN_POINT('Ctrl Pts',(57.4516131939078,-6.1117660954725,1.01987337997304));
#26238=CARTESIAN_POINT('Ctrl Pts',(58.0042447728553,-5.86054393090788,-2.0119272727519));
#26239=CARTESIAN_POINT('Ctrl Pts',(58.5568763518026,-4.1966230145796,-4.55874783141676));
#26240=CARTESIAN_POINT('Ctrl Pts',(59.1095079307501,-1.52109563915542,-6.00667083944875));
#26241=CARTESIAN_POINT('Ctrl Pts',(59.6621395096973,1.52109563915524,-6.00667083944942));
#26242=CARTESIAN_POINT('Ctrl Pts',(60.2147710886447,4.1966230145802,-4.55874783141572));
#26243=CARTESIAN_POINT('Ctrl Pts',(60.7674026675922,5.86054393090647,-2.01192727275395));
#26244=CARTESIAN_POINT('Ctrl Pts',(61.3200342465394,6.11176609547552,1.01987337997724));
#26245=CARTESIAN_POINT('Ctrl Pts',(61.8726658254869,4.88973177804935,3.80583100722426));
#26246=CARTESIAN_POINT('Ctrl Pts',(62.4252974044342,2.48901540302145,5.67438356482389));
#26247=CARTESIAN_POINT('Ctrl Pts',(62.9779289833816,-0.511684351495617,
6.17511179177572));
#26248=CARTESIAN_POINT('Ctrl Pts',(63.5305605623289,-3.38904131498585,5.18731389860973));
#26249=CARTESIAN_POINT('Ctrl Pts',(64.0831921412763,-5.44946140533107,2.94910103406098));
#26250=CARTESIAN_POINT('Ctrl Pts',(64.6358237202237,-6.19627521287463,3.62109504307536E-10));
#26251=CARTESIAN_POINT('Ctrl Pts',(65.188455299171,-5.44946140575937,-2.94910103499479));
#26252=CARTESIAN_POINT('Ctrl Pts',(65.7410868781184,-3.38904131388132,-5.18731389692575));
#26253=CARTESIAN_POINT('Ctrl Pts',(66.2937184570658,-0.511684353915733,
-6.17511179518466));
#26254=CARTESIAN_POINT('Ctrl Pts',(66.8463500360131,2.48901540815811,-5.67438355771667));
#26255=CARTESIAN_POINT('Ctrl Pts',(67.3989816149605,4.88973176722276,-3.80583102214386));
#26256=CARTESIAN_POINT('Ctrl Pts',(67.9516131939078,6.11176611825917,-1.01987334860882));
#26257=CARTESIAN_POINT('Ctrl Pts',(68.5042447728553,5.86054388297712,2.01192720677863));
#26258=CARTESIAN_POINT('Ctrl Pts',(69.0568763518026,4.19662311539983,4.55874797018865));
#26259=CARTESIAN_POINT('Ctrl Pts',(69.60950793075,1.52109542708419,6.00667054754813));
#26260=CARTESIAN_POINT('Ctrl Pts',(70.1621395096974,-1.52109519307484,6.00667145344936));
#26261=CARTESIAN_POINT('Ctrl Pts',(70.7147710886448,-4.19662395290879,4.5587465398911));
#26262=CARTESIAN_POINT('Ctrl Pts',(71.2674026675922,-5.86054195732468,2.01192998939814));
#26263=CARTESIAN_POINT('Ctrl Pts',(71.8200342465394,-6.11177024810298,-1.01987909450272));
#26264=CARTESIAN_POINT('Ctrl Pts',(72.3726658254869,-4.88972305399822,-3.80581898848348));
#26265=CARTESIAN_POINT('Ctrl Pts',(72.9252974044342,-2.48903384632581,-5.67440885923964));
#26266=CARTESIAN_POINT('Ctrl Pts',(73.4779289833816,0.511722382884753,-6.17505868653612));
#26267=CARTESIAN_POINT('Ctrl Pts',(74.0305605623289,3.38895443893944,-5.18742673184629));
#26268=CARTESIAN_POINT('Ctrl Pts',(74.5831921412763,5.44959421336945,-2.94886771297254));
#26269=CARTESIAN_POINT('Ctrl Pts',(74.9516131939079,5.94680344913766,-0.983379197578397));
#26270=CARTESIAN_POINT('Ctrl Pts',(75.1358237202237,5.94680344913766,-8.73928057097385E-15));
#26271=CARTESIAN_POINT('Ctrl Pts',(32.9926516271063,5.64959965017094,0.));
#26272=CARTESIAN_POINT('Ctrl Pts',(33.1768621534221,5.64959965017094,0.934105498328347));
#26273=CARTESIAN_POINT('Ctrl Pts',(33.5452832060536,5.17719316068765,2.80153095913731));
#26274=CARTESIAN_POINT('Ctrl Pts',(34.097914785001,3.21956825042242,4.92810992359527));
#26275=CARTESIAN_POINT('Ctrl Pts',(34.6505463639483,0.486141746602274,5.86641986341936));
#26276=CARTESIAN_POINT('Ctrl Pts',(35.2031779428958,-2.36462122333319,5.39077403004133));
#26277=CARTESIAN_POINT('Ctrl Pts',(35.7558095218431,-4.64531700059631,3.61559300345088));
#26278=CARTESIAN_POINT('Ctrl Pts',(36.3084411007905,-5.80628073241482,0.968900224297807));
#26279=CARTESIAN_POINT('Ctrl Pts',(36.8610726797378,-5.56761023028957,-1.91136547361583));
#26280=CARTESIAN_POINT('Ctrl Pts',(37.4137042586852,-3.98686087342849,-4.33088362081724));
#26281=CARTESIAN_POINT('Ctrl Pts',(37.9663358376326,-1.44506518185627,-5.7064353192738));
#26282=CARTESIAN_POINT('Ctrl Pts',(38.5189674165799,1.445065386745,-5.7064346943363));
#26283=CARTESIAN_POINT('Ctrl Pts',(39.0715989955273,3.98686014014099,-4.33088460750931));
#26284=CARTESIAN_POINT('Ctrl Pts',(39.6242305744747,5.56761191630958,-1.91136355401326));
#26285=CARTESIAN_POINT('Ctrl Pts',(40.1768621534221,5.80627711649786,0.968896260552868));
#26286=CARTESIAN_POINT('Ctrl Pts',(40.7294937323694,4.64532462952802,3.61560130546583));
#26287=CARTESIAN_POINT('Ctrl Pts',(41.2821253113168,2.36460507965162,5.39075658079754));
#26288=CARTESIAN_POINT('Ctrl Pts',(41.8347568902642,-0.486108450041791,
5.86645653965694));
#26289=CARTESIAN_POINT('Ctrl Pts',(42.3873884692115,-3.21964431445548,4.92803248756168));
#26290=CARTESIAN_POINT('Ctrl Pts',(42.9400200481589,-5.17707687994863,2.80169390094401));
#26291=CARTESIAN_POINT('Ctrl Pts',(43.4926516271062,-5.88656213122846,-2.49796196989472E-10));
#26292=CARTESIAN_POINT('Ctrl Pts',(44.0452832060537,-5.17707687957364,-2.80169390029981));
#26293=CARTESIAN_POINT('Ctrl Pts',(44.597914785001,-3.21964431542256,-4.92803248872338));
#26294=CARTESIAN_POINT('Ctrl Pts',(45.1505463639484,-0.486108447922835,
-5.86645653730528));
#26295=CARTESIAN_POINT('Ctrl Pts',(45.7031779428957,2.36460507515419,-5.39075658570046));
#26296=CARTESIAN_POINT('Ctrl Pts',(46.2558095218431,4.64532463900732,-3.61560129517351));
#26297=CARTESIAN_POINT('Ctrl Pts',(46.8084411007904,5.80627709654946,-0.968896282192427));
#26298=CARTESIAN_POINT('Ctrl Pts',(47.3610726797379,5.5676119582745,1.91136359952644));
#26299=CARTESIAN_POINT('Ctrl Pts',(47.9137042586852,3.98686005186758,4.33088451177657));
#26300=CARTESIAN_POINT('Ctrl Pts',(48.4663358376326,1.44506557242546,5.70643489570486));
#26301=CARTESIAN_POINT('Ctrl Pts',(49.0189674165799,-1.4450655724256,5.7064348957044));
#26302=CARTESIAN_POINT('Ctrl Pts',(49.5715989955273,-3.98686005186705,4.3308845117773));
#26303=CARTESIAN_POINT('Ctrl Pts',(50.1242305744747,-5.56761195827573,1.91136359952503));
#26304=CARTESIAN_POINT('Ctrl Pts',(50.6768621534221,-5.80627709654682,-0.968896282189531));
#26305=CARTESIAN_POINT('Ctrl Pts',(51.2294937323694,-4.6453246390129,-3.61560129517959));
#26306=CARTESIAN_POINT('Ctrl Pts',(51.7821253113168,-2.36460507514243,-5.3907565856877));
#26307=CARTESIAN_POINT('Ctrl Pts',(52.3347568902641,0.486108447898087,-5.86645653733213));
#26308=CARTESIAN_POINT('Ctrl Pts',(52.8873884692115,3.21964431547462,-4.92803248866692));
#26309=CARTESIAN_POINT('Ctrl Pts',(53.4400200481589,5.17707687946413,-2.80169390041857));
#26310=CARTESIAN_POINT('Ctrl Pts',(53.9926516271062,5.88656213145879,-3.62063508832155E-15));
#26311=CARTESIAN_POINT('Ctrl Pts',(54.5452832060537,5.17707687946413,2.80169390041857));
#26312=CARTESIAN_POINT('Ctrl Pts',(55.0979147850009,3.21964431547461,4.92803248866692));
#26313=CARTESIAN_POINT('Ctrl Pts',(55.6505463639484,0.486108447898084,5.86645653733212));
#26314=CARTESIAN_POINT('Ctrl Pts',(56.2031779428957,-2.36460507514244,5.3907565856877));
#26315=CARTESIAN_POINT('Ctrl Pts',(56.7558095218431,-4.64532463901291,3.61560129517958));
#26316=CARTESIAN_POINT('Ctrl Pts',(57.3084411007904,-5.80627709654682,0.968896282189525));
#26317=CARTESIAN_POINT('Ctrl Pts',(57.8610726797378,-5.56761195827573,-1.91136359952503));
#26318=CARTESIAN_POINT('Ctrl Pts',(58.4137042586852,-3.98686005186705,-4.3308845117773));
#26319=CARTESIAN_POINT('Ctrl Pts',(58.9663358376325,-1.44506557242561,-5.7064348957044));
#26320=CARTESIAN_POINT('Ctrl Pts',(59.51896741658,1.44506557242545,-5.70643489570486));
#26321=CARTESIAN_POINT('Ctrl Pts',(60.0715989955273,3.98686005186758,-4.33088451177658));
#26322=CARTESIAN_POINT('Ctrl Pts',(60.6242305744747,5.5676119582745,-1.91136359952644));
#26323=CARTESIAN_POINT('Ctrl Pts',(61.176862153422,5.80627709654946,0.968896282192422));
#26324=CARTESIAN_POINT('Ctrl Pts',(61.7294937323694,4.64532463900732,3.61560129517351));
#26325=CARTESIAN_POINT('Ctrl Pts',(62.2821253113167,2.36460507515419,5.39075658570046));
#26326=CARTESIAN_POINT('Ctrl Pts',(62.8347568902642,-0.486108447922834,
5.86645653730528));
#26327=CARTESIAN_POINT('Ctrl Pts',(63.3873884692115,-3.21964431542255,4.92803248872338));
#26328=CARTESIAN_POINT('Ctrl Pts',(63.9400200481589,-5.17707687957363,2.80169390029982));
#26329=CARTESIAN_POINT('Ctrl Pts',(64.4926516271063,-5.88656213122846,2.49803438259616E-10));
#26330=CARTESIAN_POINT('Ctrl Pts',(65.0452832060536,-5.17707687994864,-2.80169390094401));
#26331=CARTESIAN_POINT('Ctrl Pts',(65.597914785001,-3.21964431445548,-4.92803248756169));
#26332=CARTESIAN_POINT('Ctrl Pts',(66.1505463639484,-0.486108450041783,
-5.86645653965694));
#26333=CARTESIAN_POINT('Ctrl Pts',(66.7031779428957,2.36460507965163,-5.39075658079754));
#26334=CARTESIAN_POINT('Ctrl Pts',(67.255809521843,4.64532462952802,-3.61560130546582));
#26335=CARTESIAN_POINT('Ctrl Pts',(67.8084411007905,5.80627711649786,-0.96889626055287));
#26336=CARTESIAN_POINT('Ctrl Pts',(68.3610726797379,5.56761191630958,1.91136355401326));
#26337=CARTESIAN_POINT('Ctrl Pts',(68.9137042586851,3.98686014014099,4.33088460750931));
#26338=CARTESIAN_POINT('Ctrl Pts',(69.4663358376326,1.44506538674499,5.7064346943363));
#26339=CARTESIAN_POINT('Ctrl Pts',(70.0189674165799,-1.44506518185629,5.7064353192738));
#26340=CARTESIAN_POINT('Ctrl Pts',(70.5715989955273,-3.98686087342849,4.33088362081724));
#26341=CARTESIAN_POINT('Ctrl Pts',(71.1242305744747,-5.56761023028957,1.91136547361582));
#26342=CARTESIAN_POINT('Ctrl Pts',(71.6768621534221,-5.80628073241483,-0.968900224297809));
#26343=CARTESIAN_POINT('Ctrl Pts',(72.2294937323694,-4.64531700059631,-3.61559300345089));
#26344=CARTESIAN_POINT('Ctrl Pts',(72.7821253113168,-2.36462122333319,-5.39077403004132));
#26345=CARTESIAN_POINT('Ctrl Pts',(73.3347568902641,0.486141746602262,-5.86641986341937));
#26346=CARTESIAN_POINT('Ctrl Pts',(73.8873884692115,3.21956825042242,-4.92810992359527));
#26347=CARTESIAN_POINT('Ctrl Pts',(74.4400200481589,5.17719316068764,-2.80153095913731));
#26348=CARTESIAN_POINT('Ctrl Pts',(74.8084411007905,5.64959965017094,-0.934105498328348));
#26349=CARTESIAN_POINT('Ctrl Pts',(74.9926516271063,5.64959965017094,-8.30251695365502E-15));
#26350=CARTESIAN_POINT('Ctrl Pts',(32.9926516271063,5.35040034982906,0.));
#26351=CARTESIAN_POINT('Ctrl Pts',(33.1768621534221,5.35040034982906,0.884711999783592));
#26352=CARTESIAN_POINT('Ctrl Pts',(33.5452832060536,4.90303992219514,2.65314027768598));
#26353=CARTESIAN_POINT('Ctrl Pts',(34.097914785001,3.04907159007201,4.66715881783104));
#26354=CARTESIAN_POINT('Ctrl Pts',(34.6505463639483,0.460399720877627,5.55575434845313));
#26355=CARTESIAN_POINT('Ctrl Pts',(35.2031779428958,-2.23940312125801,5.10530860391639));
#26356=CARTESIAN_POINT('Ctrl Pts',(35.7558095218431,-4.39932305117563,3.42412678374845));
#26357=CARTESIAN_POINT('Ctrl Pts',(36.3084411007905,-5.49880832246205,0.917592835722961));
#26358=CARTESIAN_POINT('Ctrl Pts',(36.8610726797378,-5.272776384942,-1.81014920900501));
#26359=CARTESIAN_POINT('Ctrl Pts',(37.4137042586852,-3.77573601188937,-4.10154073270038));
#26360=CARTESIAN_POINT('Ctrl Pts',(37.9663358376326,-1.36854148671349,-5.40425015093622));
#26361=CARTESIAN_POINT('Ctrl Pts',(38.5189674165799,1.36854169117612,-5.40424941809581));
#26362=CARTESIAN_POINT('Ctrl Pts',(39.0715989955273,3.77573528012686,-4.1015418897575));
#26363=CARTESIAN_POINT('Ctrl Pts',(39.6242305744747,5.27277806745566,-1.81014695796662));
#26364=CARTESIAN_POINT('Ctrl Pts',(40.1768621534221,5.49880471406498,0.917588187532836));
#26365=CARTESIAN_POINT('Ctrl Pts',(40.7294937323694,4.39933066424171,3.42413651873231));
#26366=CARTESIAN_POINT('Ctrl Pts',(41.2821253113168,2.23938701114991,5.10528813768847));
#26367=CARTESIAN_POINT('Ctrl Pts',(41.8347568902642,-0.460366493562869,
5.55579732502866));
#26368=CARTESIAN_POINT('Ctrl Pts',(42.3873884692115,-3.04914749591728,4.66706767925751));
#26369=CARTESIAN_POINT('Ctrl Pts',(42.9400200481589,-4.90292388328124,2.65332971861579));
#26370=CARTESIAN_POINT('Ctrl Pts',(43.4926516271062,-5.57483822100387,-2.9292627494233E-10));
#26371=CARTESIAN_POINT('Ctrl Pts',(44.0452832060537,-4.90292388290702,-2.65332971786037));
#26372=CARTESIAN_POINT('Ctrl Pts',(44.597914785001,-3.04914749688235,-4.66706768061979));
#26373=CARTESIAN_POINT('Ctrl Pts',(45.1505463639484,-0.460366491448323,
-5.55579732227095));
#26374=CARTESIAN_POINT('Ctrl Pts',(45.7031779428957,2.23938700666183,-5.10528814343794));
#26375=CARTESIAN_POINT('Ctrl Pts',(46.2558095218431,4.3993306737013,-3.4241365066629));
#26376=CARTESIAN_POINT('Ctrl Pts',(46.8084411007904,5.49880469415807,-0.917588212908723));
#26377=CARTESIAN_POINT('Ctrl Pts',(47.3610726797379,5.2727781093333,1.81014701133818));
#26378=CARTESIAN_POINT('Ctrl Pts',(47.9137042586852,3.77573519203703,4.10154177749537));
#26379=CARTESIAN_POINT('Ctrl Pts',(48.4663358376326,1.36854187647043,5.40424965423309));
#26380=CARTESIAN_POINT('Ctrl Pts',(49.0189674165799,-1.36854187647057,5.40424965423255));
#26381=CARTESIAN_POINT('Ctrl Pts',(49.5715989955273,-3.7757351920365,4.10154177749621));
#26382=CARTESIAN_POINT('Ctrl Pts',(50.1242305744747,-5.27277810933453,1.81014701133654));
#26383=CARTESIAN_POINT('Ctrl Pts',(50.6768621534221,-5.49880469415544,-0.917588212905327));
#26384=CARTESIAN_POINT('Ctrl Pts',(51.2294937323694,-4.39933067370686,-3.42413650667002));
#26385=CARTESIAN_POINT('Ctrl Pts',(51.7821253113168,-2.23938700665009,-5.10528814342298));
#26386=CARTESIAN_POINT('Ctrl Pts',(52.3347568902641,0.460366491423626,-5.55579732230242));
#26387=CARTESIAN_POINT('Ctrl Pts',(52.8873884692115,3.0491474969343,-4.66706768055358));
#26388=CARTESIAN_POINT('Ctrl Pts',(53.4400200481589,4.90292388279774,-2.65332971799963));
#26389=CARTESIAN_POINT('Ctrl Pts',(53.9926516271062,5.57483822123373,-6.57078219732429E-15));
#26390=CARTESIAN_POINT('Ctrl Pts',(54.5452832060537,4.90292388279775,2.65332971799963));
#26391=CARTESIAN_POINT('Ctrl Pts',(55.0979147850009,3.0491474969343,4.66706768055358));
#26392=CARTESIAN_POINT('Ctrl Pts',(55.6505463639484,0.460366491423622,5.55579732230243));
#26393=CARTESIAN_POINT('Ctrl Pts',(56.2031779428957,-2.2393870066501,5.10528814342297));
#26394=CARTESIAN_POINT('Ctrl Pts',(56.7558095218432,-4.39933067370687,3.42413650667002));
#26395=CARTESIAN_POINT('Ctrl Pts',(57.3084411007904,-5.49880469415543,0.917588212905322));
#26396=CARTESIAN_POINT('Ctrl Pts',(57.8610726797378,-5.27277810933453,-1.81014701133654));
#26397=CARTESIAN_POINT('Ctrl Pts',(58.4137042586852,-3.7757351920365,-4.10154177749621));
#26398=CARTESIAN_POINT('Ctrl Pts',(58.9663358376325,-1.36854187647058,-5.40424965423255));
#26399=CARTESIAN_POINT('Ctrl Pts',(59.51896741658,1.36854187647042,-5.40424965423309));
#26400=CARTESIAN_POINT('Ctrl Pts',(60.0715989955273,3.77573519203703,-4.10154177749537));
#26401=CARTESIAN_POINT('Ctrl Pts',(60.6242305744747,5.2727781093333,-1.81014701133819));
#26402=CARTESIAN_POINT('Ctrl Pts',(61.176862153422,5.49880469415808,0.917588212908717));
#26403=CARTESIAN_POINT('Ctrl Pts',(61.7294937323694,4.39933067370129,3.4241365066629));
#26404=CARTESIAN_POINT('Ctrl Pts',(62.2821253113167,2.23938700666183,5.10528814343794));
#26405=CARTESIAN_POINT('Ctrl Pts',(62.8347568902642,-0.460366491448322,
5.55579732227095));
#26406=CARTESIAN_POINT('Ctrl Pts',(63.3873884692115,-3.04914749688234,4.66706768061979));
#26407=CARTESIAN_POINT('Ctrl Pts',(63.9400200481589,-4.90292388290702,2.65332971786038));
#26408=CARTESIAN_POINT('Ctrl Pts',(64.4926516271063,-5.57483822100388,2.92934052602853E-10));
#26409=CARTESIAN_POINT('Ctrl Pts',(65.0452832060536,-4.90292388328124,-2.65332971861579));
#26410=CARTESIAN_POINT('Ctrl Pts',(65.597914785001,-3.04914749591728,-4.66706767925751));
#26411=CARTESIAN_POINT('Ctrl Pts',(66.1505463639483,-0.460366493562863,
-5.55579732502866));
#26412=CARTESIAN_POINT('Ctrl Pts',(66.7031779428957,2.23938701114991,-5.10528813768846));
#26413=CARTESIAN_POINT('Ctrl Pts',(67.2558095218431,4.39933066424171,-3.4241365187323));
#26414=CARTESIAN_POINT('Ctrl Pts',(67.8084411007905,5.49880471406499,-0.917588187532837));
#26415=CARTESIAN_POINT('Ctrl Pts',(68.3610726797379,5.27277806745566,1.81014695796662));
#26416=CARTESIAN_POINT('Ctrl Pts',(68.9137042586851,3.77573528012686,4.1015418897575));
#26417=CARTESIAN_POINT('Ctrl Pts',(69.4663358376326,1.36854169117611,5.40424941809582));
#26418=CARTESIAN_POINT('Ctrl Pts',(70.0189674165799,-1.36854148671351,5.40425015093621));
#26419=CARTESIAN_POINT('Ctrl Pts',(70.5715989955273,-3.77573601188937,4.10154073270038));
#26420=CARTESIAN_POINT('Ctrl Pts',(71.1242305744747,-5.272776384942,1.81014920900501));
#26421=CARTESIAN_POINT('Ctrl Pts',(71.6768621534221,-5.49880832246205,-0.917592835722964));
#26422=CARTESIAN_POINT('Ctrl Pts',(72.2294937323694,-4.39932305117562,-3.42412678374846));
#26423=CARTESIAN_POINT('Ctrl Pts',(72.7821253113168,-2.23940312125801,-5.10530860391638));
#26424=CARTESIAN_POINT('Ctrl Pts',(73.3347568902641,0.460399720877618,-5.55575434845314));
#26425=CARTESIAN_POINT('Ctrl Pts',(73.8873884692115,3.04907159007201,-4.66715881783104));
#26426=CARTESIAN_POINT('Ctrl Pts',(74.4400200481589,4.90303992219514,-2.65314027768598));
#26427=CARTESIAN_POINT('Ctrl Pts',(74.8084411007905,5.35040034982906,-0.884711999783593));
#26428=CARTESIAN_POINT('Ctrl Pts',(74.9926516271063,5.35040034982906,-7.86282079509004E-15));
#26429=CARTESIAN_POINT('Ctrl Pts',(33.1358791011789,5.05215470582044,0.));
#26430=CARTESIAN_POINT('Ctrl Pts',(33.3200896274947,5.05215470582044,0.835439667818526));
#26431=CARTESIAN_POINT('Ctrl Pts',(33.6885106801263,4.62974731329617,2.50523368528442));
#26432=CARTESIAN_POINT('Ctrl Pts',(34.2411422590737,2.87911375329489,4.40702109952745));
#26433=CARTESIAN_POINT('Ctrl Pts',(34.793773838021,0.43473796291613,5.24607120227223));
#26434=CARTESIAN_POINT('Ctrl Pts',(35.3464054169684,-2.11457900308638,4.8207403763615));
#26435=CARTESIAN_POINT('Ctrl Pts',(35.8990369959157,-4.15410404637352,3.23326447896726));
#26436=CARTESIAN_POINT('Ctrl Pts',(36.4516685748631,-5.19230421072891,0.866446616436196));
#26437=CARTESIAN_POINT('Ctrl Pts',(37.0043001538105,-4.9788711625536,-1.70925152427458));
#26438=CARTESIAN_POINT('Ctrl Pts',(37.5569317327579,-3.56527606954637,-3.87292025722597));
#26439=CARTESIAN_POINT('Ctrl Pts',(38.1095633117052,-1.29225881290354,-5.10301667120488));
#26440=CARTESIAN_POINT('Ctrl Pts',(38.6621948906526,1.29225901197644,-5.10301589795954));
#26441=CARTESIAN_POINT('Ctrl Pts',(39.2148264696,3.56527535707347,-3.87292147807751));
#26442=CARTESIAN_POINT('Ctrl Pts',(39.7674580485474,4.97887280071541,-1.70924914912885));
#26443=CARTESIAN_POINT('Ctrl Pts',(40.3200896274947,5.19230069745088,0.8664417119428));
#26444=CARTESIAN_POINT('Ctrl Pts',(40.8727212064421,4.15411145875562,3.23327475046642));
#26445=CARTESIAN_POINT('Ctrl Pts',(41.4253527853894,2.11456331764827,4.82071877979622));
#26446=CARTESIAN_POINT('Ctrl Pts',(41.9779843643368,-0.434705611488933,
5.24611653333821));
#26447=CARTESIAN_POINT('Ctrl Pts',(42.5306159432842,-2.87918765822658,4.40692478140854));
#26448=CARTESIAN_POINT('Ctrl Pts',(43.0832475222315,-4.62963433322232,2.50543281017431));
#26449=CARTESIAN_POINT('Ctrl Pts',(43.6358791011789,-5.26409608723815,-3.09079671340081E-10));
#26450=CARTESIAN_POINT('Ctrl Pts',(44.1885106801263,-4.62963433285796,-2.50543280937723));
#26451=CARTESIAN_POINT('Ctrl Pts',(44.7411422590737,-2.87918765916621,-4.40692478284593));
#26452=CARTESIAN_POINT('Ctrl Pts',(45.293773838021,-0.434705609430123,-5.24611653042846));
#26453=CARTESIAN_POINT('Ctrl Pts',(45.8464054169684,2.1145633132785,-4.82071878586269));
#26454=CARTESIAN_POINT('Ctrl Pts',(46.3990369959157,4.15411146796585,-3.23327473773157));
#26455=CARTESIAN_POINT('Ctrl Pts',(46.9516685748631,5.19230067806873,-0.866441738717781));
#26456=CARTESIAN_POINT('Ctrl Pts',(47.5043001538105,4.97887284148914,1.70924920544305));
#26457=CARTESIAN_POINT('Ctrl Pts',(48.0569317327578,3.56527527130573,3.87292135962583));
#26458=CARTESIAN_POINT('Ctrl Pts',(48.6095633117053,1.2922591923863,5.10301614711619));
#26459=CARTESIAN_POINT('Ctrl Pts',(49.1621948906526,-1.29225919238644,5.10301614711562));
#26460=CARTESIAN_POINT('Ctrl Pts',(49.7148264696,-3.56527527130521,3.87292135962672));
#26461=CARTESIAN_POINT('Ctrl Pts',(50.2674580485474,-4.97887284149034,1.70924920544131));
#26462=CARTESIAN_POINT('Ctrl Pts',(50.8200896274947,-5.19230067806616,-0.866441738714198));
#26463=CARTESIAN_POINT('Ctrl Pts',(51.3727212064421,-4.15411146797128,-3.23327473773908));
#26464=CARTESIAN_POINT('Ctrl Pts',(51.9253527853894,-2.11456331326706,-4.8207187858469));
#26465=CARTESIAN_POINT('Ctrl Pts',(52.4779843643368,0.434705609406076,-5.24611653046166));
#26466=CARTESIAN_POINT('Ctrl Pts',(53.0306159432842,2.87918765921679,-4.40692478277608));
#26467=CARTESIAN_POINT('Ctrl Pts',(53.5832475222316,4.62963433275156,-2.50543280952418));
#26468=CARTESIAN_POINT('Ctrl Pts',(54.1358791011789,5.26409608746195,-1.74326874622889E-15));
#26469=CARTESIAN_POINT('Ctrl Pts',(54.6885106801263,4.62963433275157,2.50543280952417));
#26470=CARTESIAN_POINT('Ctrl Pts',(55.2411422590736,2.87918765921679,4.40692478277608));
#26471=CARTESIAN_POINT('Ctrl Pts',(55.793773838021,0.434705609406073,5.24611653046167));
#26472=CARTESIAN_POINT('Ctrl Pts',(56.3464054169684,-2.11456331326707,4.82071878584689));
#26473=CARTESIAN_POINT('Ctrl Pts',(56.8990369959158,-4.15411146797128,3.23327473773908));
#26474=CARTESIAN_POINT('Ctrl Pts',(57.4516685748631,-5.19230067806616,0.866441738714194));
#26475=CARTESIAN_POINT('Ctrl Pts',(58.0043001538105,-4.97887284149034,-1.70924920544131));
#26476=CARTESIAN_POINT('Ctrl Pts',(58.5569317327579,-3.56527527130521,-3.87292135962672));
#26477=CARTESIAN_POINT('Ctrl Pts',(59.1095633117052,-1.29225919238644,-5.10301614711562));
#26478=CARTESIAN_POINT('Ctrl Pts',(59.6621948906526,1.29225919238629,-5.10301614711619));
#26479=CARTESIAN_POINT('Ctrl Pts',(60.2148264696,3.56527527130572,-3.87292135962584));
#26480=CARTESIAN_POINT('Ctrl Pts',(60.7674580485473,4.97887284148913,-1.70924920544305));
#26481=CARTESIAN_POINT('Ctrl Pts',(61.3200896274947,5.19230067806873,0.866441738717778));
#26482=CARTESIAN_POINT('Ctrl Pts',(61.8727212064421,4.15411146796585,3.23327473773157));
#26483=CARTESIAN_POINT('Ctrl Pts',(62.4253527853894,2.11456331327849,4.82071878586269));
#26484=CARTESIAN_POINT('Ctrl Pts',(62.9779843643369,-0.434705609430122,
5.24611653042845));
#26485=CARTESIAN_POINT('Ctrl Pts',(63.5306159432841,-2.8791876591662,4.40692478284593));
#26486=CARTESIAN_POINT('Ctrl Pts',(64.0832475222316,-4.62963433285796,2.50543280937724));
#26487=CARTESIAN_POINT('Ctrl Pts',(64.6358791011789,-5.26409608723815,3.09085705731855E-10));
#26488=CARTESIAN_POINT('Ctrl Pts',(65.1885106801263,-4.62963433322232,-2.50543281017431));
#26489=CARTESIAN_POINT('Ctrl Pts',(65.7411422590737,-2.87918765822658,-4.40692478140855));
#26490=CARTESIAN_POINT('Ctrl Pts',(66.293773838021,-0.434705611488927,-5.24611653333821));
#26491=CARTESIAN_POINT('Ctrl Pts',(66.8464054169685,2.11456331764827,-4.82071877979622));
#26492=CARTESIAN_POINT('Ctrl Pts',(67.3990369959157,4.15411145875562,-3.23327475046641));
#26493=CARTESIAN_POINT('Ctrl Pts',(67.9516685748631,5.19230069745088,-0.866441711942802));
#26494=CARTESIAN_POINT('Ctrl Pts',(68.5043001538105,4.97887280071541,1.70924914912885));
#26495=CARTESIAN_POINT('Ctrl Pts',(69.0569317327578,3.56527535707346,3.87292147807751));
#26496=CARTESIAN_POINT('Ctrl Pts',(69.6095633117052,1.29225901197643,5.10301589795954));
#26497=CARTESIAN_POINT('Ctrl Pts',(70.1621948906526,-1.29225881290355,5.10301667120488));
#26498=CARTESIAN_POINT('Ctrl Pts',(70.7148264696,-3.56527606954638,3.87292025722596));
#26499=CARTESIAN_POINT('Ctrl Pts',(71.2674580485474,-4.9788711625536,1.70925152427458));
#26500=CARTESIAN_POINT('Ctrl Pts',(71.8200896274948,-5.19230421072891,-0.866446616436202));
#26501=CARTESIAN_POINT('Ctrl Pts',(72.3727212064421,-4.15410404637352,-3.23326447896727));
#26502=CARTESIAN_POINT('Ctrl Pts',(72.9253527853895,-2.11457900308638,-4.82074037636149));
#26503=CARTESIAN_POINT('Ctrl Pts',(73.4779843643368,0.434737962916119,-5.24607120227223));
#26504=CARTESIAN_POINT('Ctrl Pts',(74.0306159432842,2.87911375329489,-4.40702109952745));
#26505=CARTESIAN_POINT('Ctrl Pts',(74.5832475222315,4.62974731329617,-2.50523368528442));
#26506=CARTESIAN_POINT('Ctrl Pts',(74.9516685748631,5.05215470582044,-0.835439667818527));
#26507=CARTESIAN_POINT('Ctrl Pts',(75.1358791011789,5.05215470582044,-7.4245261071363E-15));
#26508=CARTESIAN_POINT('Ctrl Pts',(33.6197755720781,4.94250112032697,0.));
#26509=CARTESIAN_POINT('Ctrl Pts',(33.8039860983939,4.94250112032697,0.817139076837683));
#26510=CARTESIAN_POINT('Ctrl Pts',(34.1724071510254,4.52920068974087,2.45091075495199));
#26511=CARTESIAN_POINT('Ctrl Pts',(34.7250387299729,2.81660319447189,4.31128469373266));
#26512=CARTESIAN_POINT('Ctrl Pts',(35.2776703089202,0.42529402211631,5.13217251323705));
#26513=CARTESIAN_POINT('Ctrl Pts',(35.8303018878676,-2.06865974125642,4.71605075332317));
#26514=CARTESIAN_POINT('Ctrl Pts',(36.3829334668149,-4.06389977762583,3.16305923338873));
#26515=CARTESIAN_POINT('Ctrl Pts',(36.9355650457623,-5.07955447125059,0.847630025952494));
#26516=CARTESIAN_POINT('Ctrl Pts',(37.4881966247097,-4.87075665964084,-1.67213470664358));
#26517=CARTESIAN_POINT('Ctrl Pts',(38.0408282036571,-3.48785707483957,-3.78882139657513));
#26518=CARTESIAN_POINT('Ctrl Pts',(38.5934597826044,-1.26419784346094,-4.9922059811041));
#26519=CARTESIAN_POINT('Ctrl Pts',(39.1460913615518,1.26419801522272,-4.99220553559825));
#26520=CARTESIAN_POINT('Ctrl Pts',(39.6987229404992,3.48785646011191,-3.78882209996813));
#26521=CARTESIAN_POINT('Ctrl Pts',(40.2513545194465,4.87075807306072,-1.67213333819149));
#26522=CARTESIAN_POINT('Ctrl Pts',(40.8039860983939,5.07955143996455,0.847627200316705));
#26523=CARTESIAN_POINT('Ctrl Pts',(41.3566176773413,4.06390617309189,3.16306515207384));
#26524=CARTESIAN_POINT('Ctrl Pts',(41.9092492562886,2.06864620772757,4.71603831708452));
#26525=CARTESIAN_POINT('Ctrl Pts',(42.461880835236,-0.425266109030922,5.13219868216793));
#26526=CARTESIAN_POINT('Ctrl Pts',(43.0145124141834,-2.81666696027288,4.3112297296128));
#26527=CARTESIAN_POINT('Ctrl Pts',(43.5671439931307,-4.52910320957627,2.45102808648086));
#26528=CARTESIAN_POINT('Ctrl Pts',(44.1197755720781,-5.14978781662001,-1.78074231939325E-10));
#26529=CARTESIAN_POINT('Ctrl Pts',(44.6724071510254,-4.5291032092619,-2.45102808602162));
#26530=CARTESIAN_POINT('Ctrl Pts',(45.2250387299728,-2.8166669610836,-4.31122973044095));
#26531=CARTESIAN_POINT('Ctrl Pts',(45.7776703089202,-0.425266107254567,
-5.13219868049148));
#26532=CARTESIAN_POINT('Ctrl Pts',(46.3303018878675,2.06864620395729,-4.71603832057972));
#26533=CARTESIAN_POINT('Ctrl Pts',(46.882933466815,4.06390618103855,-3.16306514473666));
#26534=CARTESIAN_POINT('Ctrl Pts',(47.4355650457623,5.07955142324146,-0.847627215743122));
#26535=CARTESIAN_POINT('Ctrl Pts',(47.9881966247097,4.87075810824064,1.67213337063694));
#26536=CARTESIAN_POINT('Ctrl Pts',(48.540828203657,3.48785638611078,3.78882203172213));
#26537=CARTESIAN_POINT('Ctrl Pts',(49.0934597826044,1.26419817088188,4.99220567914997));
#26538=CARTESIAN_POINT('Ctrl Pts',(49.6460913615518,-1.264198170882,4.99220567914965));
#26539=CARTESIAN_POINT('Ctrl Pts',(50.1987229404991,-3.48785638611033,3.78882203172264));
#26540=CARTESIAN_POINT('Ctrl Pts',(50.7513545194465,-4.87075810824168,1.67213337063594));
#26541=CARTESIAN_POINT('Ctrl Pts',(51.3039860983939,-5.07955142323925,-0.847627215741061));
#26542=CARTESIAN_POINT('Ctrl Pts',(51.8566176773412,-4.06390618104323,-3.16306514474098));
#26543=CARTESIAN_POINT('Ctrl Pts',(52.4092492562886,-2.06864620394743,-4.71603832057063));
#26544=CARTESIAN_POINT('Ctrl Pts',(52.961880835236,0.425266107233821,-5.13219868051061));
#26545=CARTESIAN_POINT('Ctrl Pts',(53.5145124141833,2.81666696112724,-4.31122973040071));
#26546=CARTESIAN_POINT('Ctrl Pts',(54.0671439931307,4.5291032091701,-2.45102808610628));
#26547=CARTESIAN_POINT('Ctrl Pts',(54.6197755720781,5.14978781681311,-5.90029421800548E-15));
#26548=CARTESIAN_POINT('Ctrl Pts',(55.1724071510255,4.52910320917011,2.45102808610628));
#26549=CARTESIAN_POINT('Ctrl Pts',(55.7250387299728,2.81666696112724,4.3112297304007));
#26550=CARTESIAN_POINT('Ctrl Pts',(56.2776703089202,0.425266107233817,5.13219868051062));
#26551=CARTESIAN_POINT('Ctrl Pts',(56.8303018878676,-2.06864620394744,4.71603832057062));
#26552=CARTESIAN_POINT('Ctrl Pts',(57.3829334668149,-4.06390618104323,3.16306514474098));
#26553=CARTESIAN_POINT('Ctrl Pts',(57.9355650457622,-5.07955142323925,0.847627215741054));
#26554=CARTESIAN_POINT('Ctrl Pts',(58.4881966247097,-4.87075810824168,-1.67213337063594));
#26555=CARTESIAN_POINT('Ctrl Pts',(59.0408282036571,-3.48785638611033,-3.78882203172264));
#26556=CARTESIAN_POINT('Ctrl Pts',(59.5934597826044,-1.26419817088201,-4.99220567914965));
#26557=CARTESIAN_POINT('Ctrl Pts',(60.1460913615518,1.26419817088187,-4.99220567914997));
#26558=CARTESIAN_POINT('Ctrl Pts',(60.6987229404992,3.48785638611077,-3.78882203172213));
#26559=CARTESIAN_POINT('Ctrl Pts',(61.2513545194465,4.87075810824064,-1.67213337063695));
#26560=CARTESIAN_POINT('Ctrl Pts',(61.8039860983939,5.07955142324146,0.847627215743118));
#26561=CARTESIAN_POINT('Ctrl Pts',(62.3566176773412,4.06390618103855,3.16306514473665));
#26562=CARTESIAN_POINT('Ctrl Pts',(62.9092492562886,2.06864620395729,4.71603832057972));
#26563=CARTESIAN_POINT('Ctrl Pts',(63.461880835236,-0.425266107254564,5.13219868049148));
#26564=CARTESIAN_POINT('Ctrl Pts',(64.0145124141834,-2.8166669610836,4.31122973044095));
#26565=CARTESIAN_POINT('Ctrl Pts',(64.5671439931307,-4.5291032092619,2.45102808602162));
#26566=CARTESIAN_POINT('Ctrl Pts',(65.1197755720782,-5.14978781662001,1.78081473209479E-10));
#26567=CARTESIAN_POINT('Ctrl Pts',(65.6724071510254,-4.52910320957627,-2.45102808648086));
#26568=CARTESIAN_POINT('Ctrl Pts',(66.2250387299728,-2.81666696027288,-4.3112297296128));
#26569=CARTESIAN_POINT('Ctrl Pts',(66.7776703089202,-0.425266109030917,
-5.13219868216794));
#26570=CARTESIAN_POINT('Ctrl Pts',(67.3303018878675,2.06864620772757,-4.71603831708452));
#26571=CARTESIAN_POINT('Ctrl Pts',(67.8829334668149,4.06390617309189,-3.16306515207384));
#26572=CARTESIAN_POINT('Ctrl Pts',(68.4355650457623,5.07955143996455,-0.847627200316705));
#26573=CARTESIAN_POINT('Ctrl Pts',(68.9881966247097,4.87075807306072,1.67213333819149));
#26574=CARTESIAN_POINT('Ctrl Pts',(69.540828203657,3.48785646011191,3.78882209996812));
#26575=CARTESIAN_POINT('Ctrl Pts',(70.0934597826044,1.26419801522272,4.99220553559826));
#26576=CARTESIAN_POINT('Ctrl Pts',(70.6460913615518,-1.26419784346096,4.99220598110409));
#26577=CARTESIAN_POINT('Ctrl Pts',(71.1987229404992,-3.48785707483957,3.78882139657512));
#26578=CARTESIAN_POINT('Ctrl Pts',(71.7513545194465,-4.87075665964084,1.67213470664358));
#26579=CARTESIAN_POINT('Ctrl Pts',(72.3039860983939,-5.0795544712506,-0.847630025952498));
#26580=CARTESIAN_POINT('Ctrl Pts',(72.8566176773413,-4.06389977762583,-3.16305923338874));
#26581=CARTESIAN_POINT('Ctrl Pts',(73.4092492562886,-2.06865974125642,-4.71605075332316));
#26582=CARTESIAN_POINT('Ctrl Pts',(73.961880835236,0.425294022116303,-5.13217251323706));
#26583=CARTESIAN_POINT('Ctrl Pts',(74.5145124141834,2.81660319447188,-4.31128469373267));
#26584=CARTESIAN_POINT('Ctrl Pts',(75.0671439931307,4.52920068974087,-2.45091075495198));
#26585=CARTESIAN_POINT('Ctrl Pts',(75.4355650457623,4.94250112032697,-0.817139076837684));
#26586=CARTESIAN_POINT('Ctrl Pts',(75.6197755720781,4.94250112032697,-7.26338181214876E-15));
#26587=CARTESIAN_POINT('Ctrl Pts',(33.9441734627902,5.19996900808372,0.));
#26588=CARTESIAN_POINT('Ctrl Pts',(34.128383989106,5.19996900808372,0.859814026526804));
#26589=CARTESIAN_POINT('Ctrl Pts',(34.4968050417376,4.76517797451894,2.57855204094631));
#26590=CARTESIAN_POINT('Ctrl Pts',(35.0494366206849,2.96334119934827,4.53592553639668));
#26591=CARTESIAN_POINT('Ctrl Pts',(35.6020681996323,0.447454012565768,5.39954421798947));
#26592=CARTESIAN_POINT('Ctrl Pts',(36.1546997785797,-2.17643695412734,4.96176002173633));
#26593=CARTESIAN_POINT('Ctrl Pts',(36.707331357527,-4.27562619453865,3.32785024601096));
#26594=CARTESIAN_POINT('Ctrl Pts',(37.2599629364744,-5.34419675899476,0.891792351082074));
#26595=CARTESIAN_POINT('Ctrl Pts',(37.8125945154218,-5.12452030784397,-1.75925261524249));
#26596=CARTESIAN_POINT('Ctrl Pts',(38.3652260943691,-3.66957259079425,-3.98621664555567));
#26597=CARTESIAN_POINT('Ctrl Pts',(38.9178576733165,-1.33006183535942,-5.25229733317933));
#26598=CARTESIAN_POINT('Ctrl Pts',(39.4704892522639,1.33006203085693,-5.25229666444782));
#26599=CARTESIAN_POINT('Ctrl Pts',(40.0231208312112,3.6695718911175,-3.98621770139316));
#26600=CARTESIAN_POINT('Ctrl Pts',(40.5757524101586,5.12452191658404,-1.75925056112342));
#26601=CARTESIAN_POINT('Ctrl Pts',(41.1283839891059,5.34419330881595,0.891788109530082));
#26602=CARTESIAN_POINT('Ctrl Pts',(41.6810155680534,4.27563347379279,3.32785912949593));
#26603=CARTESIAN_POINT('Ctrl Pts',(42.2336471470007,2.17642155040303,4.96174134693238));
#26604=CARTESIAN_POINT('Ctrl Pts',(42.7862787259481,-0.44742224217709,5.39958344300911));
#26605=CARTESIAN_POINT('Ctrl Pts',(43.3389103048954,-2.96341377693166,4.53584245342762));
#26606=CARTESIAN_POINT('Ctrl Pts',(43.8915418838428,-4.76506702359125,2.57872531691644));
#26607=CARTESIAN_POINT('Ctrl Pts',(44.4441734627902,-5.41808896103925,-2.67301766495115E-10));
#26608=CARTESIAN_POINT('Ctrl Pts',(44.9968050417375,-4.76506702323344,-2.5787253162271));
#26609=CARTESIAN_POINT('Ctrl Pts',(45.5494366206849,-2.96341377785441,-4.53584245467072));
#26610=CARTESIAN_POINT('Ctrl Pts',(46.1020681996323,-0.447422240155257,
-5.39958344049266));
#26611=CARTESIAN_POINT('Ctrl Pts',(46.6546997785796,2.17642154611174,-4.96174135217889));
#26612=CARTESIAN_POINT('Ctrl Pts',(47.207331357527,4.27563348283759,-3.32785911848237));
#26613=CARTESIAN_POINT('Ctrl Pts',(47.7599629364744,5.3441932897819,-0.891788132686083));
#26614=CARTESIAN_POINT('Ctrl Pts',(48.3125945154218,5.12452195662546,1.75925060982603));
#26615=CARTESIAN_POINT('Ctrl Pts',(48.8652260943691,3.66957180689017,3.98621759895172));
#26616=CARTESIAN_POINT('Ctrl Pts',(49.4178576733165,1.33006220802659,5.25229687992779));
#26617=CARTESIAN_POINT('Ctrl Pts',(49.9704892522639,-1.33006220802673,5.2522968799273));
#26618=CARTESIAN_POINT('Ctrl Pts',(50.5231208312112,-3.66957180688966,3.9862175989525));
#26619=CARTESIAN_POINT('Ctrl Pts',(51.0757524101586,-5.12452195662665,1.75925060982452));
#26620=CARTESIAN_POINT('Ctrl Pts',(51.628383989106,-5.34419328977938,-0.891788132682984));
#26621=CARTESIAN_POINT('Ctrl Pts',(52.1810155680533,-4.27563348284292,-3.32785911848886));
#26622=CARTESIAN_POINT('Ctrl Pts',(52.7336471470007,-2.17642154610051,-4.96174135216523));
#26623=CARTESIAN_POINT('Ctrl Pts',(53.2862787259481,0.447422240131642,-5.39958344052137));
#26624=CARTESIAN_POINT('Ctrl Pts',(53.8389103048955,2.96341377790408,-4.53584245461031));
#26625=CARTESIAN_POINT('Ctrl Pts',(54.3915418838428,4.76506702312895,-2.57872531635419));
#26626=CARTESIAN_POINT('Ctrl Pts',(54.9441734627902,5.41808896125903,-4.00057827660221E-15));
#26627=CARTESIAN_POINT('Ctrl Pts',(55.4968050417376,4.76506702312896,2.57872531635418));
#26628=CARTESIAN_POINT('Ctrl Pts',(56.0494366206849,2.96341377790408,4.5358424546103));
#26629=CARTESIAN_POINT('Ctrl Pts',(56.6020681996323,0.44742224013164,5.39958344052138));
#26630=CARTESIAN_POINT('Ctrl Pts',(57.1546997785797,-2.17642154610052,4.96174135216522));
#26631=CARTESIAN_POINT('Ctrl Pts',(57.707331357527,-4.27563348284293,3.32785911848886));
#26632=CARTESIAN_POINT('Ctrl Pts',(58.2599629364744,-5.34419328977938,0.89178813268298));
#26633=CARTESIAN_POINT('Ctrl Pts',(58.8125945154218,-5.12452195662665,-1.75925060982453));
#26634=CARTESIAN_POINT('Ctrl Pts',(59.3652260943691,-3.66957180688966,-3.9862175989525));
#26635=CARTESIAN_POINT('Ctrl Pts',(59.9178576733165,-1.33006220802674,-5.2522968799273));
#26636=CARTESIAN_POINT('Ctrl Pts',(60.4704892522639,1.33006220802658,-5.2522968799278));
#26637=CARTESIAN_POINT('Ctrl Pts',(61.0231208312112,3.66957180689017,-3.98621759895173));
#26638=CARTESIAN_POINT('Ctrl Pts',(61.5757524101587,5.12452195662546,-1.75925060982604));
#26639=CARTESIAN_POINT('Ctrl Pts',(62.128383989106,5.3441932897819,0.891788132686079));
#26640=CARTESIAN_POINT('Ctrl Pts',(62.6810155680533,4.27563348283759,3.32785911848237));
#26641=CARTESIAN_POINT('Ctrl Pts',(63.2336471470007,2.17642154611174,4.96174135217889));
#26642=CARTESIAN_POINT('Ctrl Pts',(63.7862787259481,-0.447422240155256,
5.39958344049265));
#26643=CARTESIAN_POINT('Ctrl Pts',(64.3389103048954,-2.96341377785441,4.53584245467072));
#26644=CARTESIAN_POINT('Ctrl Pts',(64.8915418838428,-4.76506702323344,2.57872531622711));
#26645=CARTESIAN_POINT('Ctrl Pts',(65.4441734627902,-5.41808896103925,2.67308784269264E-10));
#26646=CARTESIAN_POINT('Ctrl Pts',(65.9968050417376,-4.76506702359125,-2.57872531691644));
#26647=CARTESIAN_POINT('Ctrl Pts',(66.5494366206849,-2.96341377693166,-4.53584245342762));
#26648=CARTESIAN_POINT('Ctrl Pts',(67.1020681996323,-0.447422242177083,
-5.39958344300911));
#26649=CARTESIAN_POINT('Ctrl Pts',(67.6546997785796,2.17642155040303,-4.96174134693238));
#26650=CARTESIAN_POINT('Ctrl Pts',(68.2073313575271,4.27563347379279,-3.32785912949593));
#26651=CARTESIAN_POINT('Ctrl Pts',(68.7599629364744,5.34419330881595,-0.891788109530083));
#26652=CARTESIAN_POINT('Ctrl Pts',(69.3125945154218,5.12452191658404,1.75925056112342));
#26653=CARTESIAN_POINT('Ctrl Pts',(69.8652260943691,3.6695718911175,3.98621770139316));
#26654=CARTESIAN_POINT('Ctrl Pts',(70.4178576733165,1.33006203085692,5.25229666444782));
#26655=CARTESIAN_POINT('Ctrl Pts',(70.9704892522639,-1.33006183535944,5.25229733317932));
#26656=CARTESIAN_POINT('Ctrl Pts',(71.5231208312112,-3.66957259079425,3.98621664555566));
#26657=CARTESIAN_POINT('Ctrl Pts',(72.0757524101586,-5.12452030784397,1.75925261524249));
#26658=CARTESIAN_POINT('Ctrl Pts',(72.628383989106,-5.34419675899477,-0.891792351082077));
#26659=CARTESIAN_POINT('Ctrl Pts',(73.1810155680534,-4.27562619453864,-3.32785024601098));
#26660=CARTESIAN_POINT('Ctrl Pts',(73.7336471470007,-2.17643695412734,-4.96176002173632));
#26661=CARTESIAN_POINT('Ctrl Pts',(74.2862787259481,0.447454012565758,-5.39954421798947));
#26662=CARTESIAN_POINT('Ctrl Pts',(74.8389103048955,2.96334119934827,-4.53592553639669));
#26663=CARTESIAN_POINT('Ctrl Pts',(75.3915418838428,4.76517797451894,-2.5785520409463));
#26664=CARTESIAN_POINT('Ctrl Pts',(75.7599629364744,5.19996900808372,-0.859814026526805));
#26665=CARTESIAN_POINT('Ctrl Pts',(75.9441734627902,5.19996900808372,-7.6417504816982E-15));
#26666=CARTESIAN_POINT('Ctrl Pts',(33.992328768859,5.42478616651165,0.));
#26667=CARTESIAN_POINT('Ctrl Pts',(34.1765392951748,5.42478616651165,0.897005658049128));
#26668=CARTESIAN_POINT('Ctrl Pts',(34.5449603478064,4.97120383948995,2.69002843971947));
#26669=CARTESIAN_POINT('Ctrl Pts',(35.0975919267537,3.09146156820945,4.73204241007042));
#26670=CARTESIAN_POINT('Ctrl Pts',(35.6502235057011,0.46680027700504,5.63299379713529));
#26671=CARTESIAN_POINT('Ctrl Pts',(36.2028550846485,-2.27053630835485,5.1762847224297));
#26672=CARTESIAN_POINT('Ctrl Pts',(36.7554866635958,-4.46048458163846,3.47173079196878));
#26673=CARTESIAN_POINT('Ctrl Pts',(37.3081182425432,-5.57525537632878,0.930349576908284));
#26674=CARTESIAN_POINT('Ctrl Pts',(37.8607498214906,-5.34608105725119,-1.83531473574165));
#26675=CARTESIAN_POINT('Ctrl Pts',(38.4133814004379,-3.82822810044738,-4.15856233495235));
#26676=CARTESIAN_POINT('Ctrl Pts',(38.9660129793853,-1.3875676081727,-5.47938261924127));
#26677=CARTESIAN_POINT('Ctrl Pts',(39.5186445583327,1.38756781460722,-5.47938188798928));
#26678=CARTESIAN_POINT('Ctrl Pts',(40.07127613728,3.82822736162757,-4.1585634895015));
#26679=CARTESIAN_POINT('Ctrl Pts',(40.6239077162274,5.34608275599143,-1.83531248958194));
#26680=CARTESIAN_POINT('Ctrl Pts',(41.1765392951747,5.57525173313143,0.93034493879696));
#26681=CARTESIAN_POINT('Ctrl Pts',(41.7291708741222,4.46049226812687,3.471740505884));
#26682=CARTESIAN_POINT('Ctrl Pts',(42.2818024530695,2.27052004287681,5.17626430084314));
#26683=CARTESIAN_POINT('Ctrl Pts',(42.8344340320169,-0.466766729237704,
5.6330366827348));
#26684=CARTESIAN_POINT('Ctrl Pts',(43.3870656109642,-3.09153820610978,4.73195149145368));
#26685=CARTESIAN_POINT('Ctrl Pts',(43.9396971899116,-4.97108668146758,2.69021758030695));
#26686=CARTESIAN_POINT('Ctrl Pts',(44.492328768859,-5.65234229441848,-2.92291792167501E-10));
#26687=CARTESIAN_POINT('Ctrl Pts',(45.0449603478063,-4.97108668108975,-2.69021757955316));
#26688=CARTESIAN_POINT('Ctrl Pts',(45.5975919267537,-3.09153820708416,-4.731951492813));
#26689=CARTESIAN_POINT('Ctrl Pts',(46.1502235057011,-0.466766727102762,
-5.63303667998308));
#26690=CARTESIAN_POINT('Ctrl Pts',(46.7028550846484,2.27052003834545,-5.17626430658015));
#26691=CARTESIAN_POINT('Ctrl Pts',(47.2554866635958,4.46049227767768,-3.47174049384076));
#26692=CARTESIAN_POINT('Ctrl Pts',(47.8081182425432,5.57525171303253,-0.930344964117844));
#26693=CARTESIAN_POINT('Ctrl Pts',(48.3607498214906,5.34608279827294,1.83531254283782));
#26694=CARTESIAN_POINT('Ctrl Pts',(48.9133814004379,3.82822727268818,4.15856337748268));
#26695=CARTESIAN_POINT('Ctrl Pts',(49.4660129793853,1.38756800168855,5.47938212361473));
#26696=CARTESIAN_POINT('Ctrl Pts',(50.0186445583327,-1.3875680016887,5.4793821236142));
#26697=CARTESIAN_POINT('Ctrl Pts',(50.57127613728,-3.82822727268764,4.15856337748353));
#26698=CARTESIAN_POINT('Ctrl Pts',(51.1239077162274,-5.34608279827419,1.83531254283617));
#26699=CARTESIAN_POINT('Ctrl Pts',(51.6765392951748,-5.57525171302987,-0.930344964114455));
#26700=CARTESIAN_POINT('Ctrl Pts',(52.2291708741221,-4.46049227768331,-3.47174049384787));
#26701=CARTESIAN_POINT('Ctrl Pts',(52.7818024530695,-2.27052003833359,-5.17626430656522));
#26702=CARTESIAN_POINT('Ctrl Pts',(53.3344340320169,0.466766727077827,-5.63303668001448));
#26703=CARTESIAN_POINT('Ctrl Pts',(53.8870656109643,3.09153820713661,-4.73195149274695));
#26704=CARTESIAN_POINT('Ctrl Pts',(54.4396971899116,4.97108668097941,-2.69021757969212));
#26705=CARTESIAN_POINT('Ctrl Pts',(54.992328768859,5.65234229465055,-4.82192605126774E-15));
#26706=CARTESIAN_POINT('Ctrl Pts',(55.5449603478064,4.97108668097942,2.69021757969212));
#26707=CARTESIAN_POINT('Ctrl Pts',(56.0975919267537,3.09153820713661,4.73195149274694));
#26708=CARTESIAN_POINT('Ctrl Pts',(56.6502235057011,0.466766727077823,5.63303668001448));
#26709=CARTESIAN_POINT('Ctrl Pts',(57.2028550846485,-2.2705200383336,5.17626430656521));
#26710=CARTESIAN_POINT('Ctrl Pts',(57.7554866635958,-4.46049227768332,3.47174049384786));
#26711=CARTESIAN_POINT('Ctrl Pts',(58.3081182425432,-5.57525171302987,0.930344964114451));
#26712=CARTESIAN_POINT('Ctrl Pts',(58.8607498214906,-5.34608279827419,-1.83531254283618));
#26713=CARTESIAN_POINT('Ctrl Pts',(59.4133814004379,-3.82822727268764,-4.15856337748353));
#26714=CARTESIAN_POINT('Ctrl Pts',(59.9660129793853,-1.3875680016887,-5.47938212361419));
#26715=CARTESIAN_POINT('Ctrl Pts',(60.5186445583327,1.38756800168854,-5.47938212361474));
#26716=CARTESIAN_POINT('Ctrl Pts',(61.07127613728,3.82822727268818,-4.15856337748269));
#26717=CARTESIAN_POINT('Ctrl Pts',(61.6239077162275,5.34608279827295,-1.83531254283783));
#26718=CARTESIAN_POINT('Ctrl Pts',(62.1765392951748,5.57525171303254,0.93034496411784));
#26719=CARTESIAN_POINT('Ctrl Pts',(62.7291708741221,4.46049227767768,3.47174049384076));
#26720=CARTESIAN_POINT('Ctrl Pts',(63.2818024530695,2.27052003834545,5.17626430658015));
#26721=CARTESIAN_POINT('Ctrl Pts',(63.8344340320169,-0.466766727102761,
5.63303667998307));
#26722=CARTESIAN_POINT('Ctrl Pts',(64.3870656109642,-3.09153820708416,4.731951492813));
#26723=CARTESIAN_POINT('Ctrl Pts',(64.9396971899116,-4.97108668108975,2.69021757955317));
#26724=CARTESIAN_POINT('Ctrl Pts',(65.492328768859,-5.65234229441848,2.92299128423437E-10));
#26725=CARTESIAN_POINT('Ctrl Pts',(66.0449603478064,-4.97108668146758,-2.69021758030695));
#26726=CARTESIAN_POINT('Ctrl Pts',(66.5975919267537,-3.09153820610978,-4.73195149145368));
#26727=CARTESIAN_POINT('Ctrl Pts',(67.1502235057011,-0.466766729237698,
-5.6330366827348));
#26728=CARTESIAN_POINT('Ctrl Pts',(67.7028550846484,2.27052004287681,-5.17626430084314));
#26729=CARTESIAN_POINT('Ctrl Pts',(68.2554866635959,4.46049226812687,-3.471740505884));
#26730=CARTESIAN_POINT('Ctrl Pts',(68.8081182425432,5.57525173313144,-0.930344938796962));
#26731=CARTESIAN_POINT('Ctrl Pts',(69.3607498214906,5.34608275599143,1.83531248958194));
#26732=CARTESIAN_POINT('Ctrl Pts',(69.9133814004379,3.82822736162757,4.15856348950149));
#26733=CARTESIAN_POINT('Ctrl Pts',(70.4660129793853,1.38756781460721,5.47938188798929));
#26734=CARTESIAN_POINT('Ctrl Pts',(71.0186445583327,-1.38756760817271,5.47938261924127));
#26735=CARTESIAN_POINT('Ctrl Pts',(71.5712761372801,-3.82822810044738,4.15856233495234));
#26736=CARTESIAN_POINT('Ctrl Pts',(72.1239077162274,-5.34608105725119,1.83531473574165));
#26737=CARTESIAN_POINT('Ctrl Pts',(72.6765392951748,-5.57525537632879,-0.930349576908287));
#26738=CARTESIAN_POINT('Ctrl Pts',(73.2291708741222,-4.46048458163846,-3.4717307919688));
#26739=CARTESIAN_POINT('Ctrl Pts',(73.7818024530695,-2.27053630835485,-5.1762847224297));
#26740=CARTESIAN_POINT('Ctrl Pts',(74.3344340320169,0.46680027700503,-5.63299379713529));
#26741=CARTESIAN_POINT('Ctrl Pts',(74.8870656109643,3.09146156820945,-4.73204241007043));
#26742=CARTESIAN_POINT('Ctrl Pts',(75.4396971899116,4.97120383948995,-2.69002843971946));
#26743=CARTESIAN_POINT('Ctrl Pts',(75.8081182425432,5.42478616651165,-0.897005658049129));
#26744=CARTESIAN_POINT('Ctrl Pts',(75.992328768859,5.42478616651165,-7.9721364178528E-15));
#26745=CARTESIAN_POINT('Ctrl Pts',(33.9921997677122,5.49976642738082,0.));
#26746=CARTESIAN_POINT('Ctrl Pts',(34.176410294028,5.49976642738082,0.909403588662882));
#26747=CARTESIAN_POINT('Ctrl Pts',(34.5448313466596,5.03991467318512,2.72720954086847));
#26748=CARTESIAN_POINT('Ctrl Pts',(35.0974629256069,3.13419106663809,4.79744756259311));
#26749=CARTESIAN_POINT('Ctrl Pts',(35.6500945045543,0.473252278446431,5.71085179682633));
#26750=CARTESIAN_POINT('Ctrl Pts',(36.2027260835017,-2.30191914515453,5.24783014539696));
#26751=CARTESIAN_POINT('Ctrl Pts',(36.755357662449,-4.52213639346893,3.51971627798693));
#26752=CARTESIAN_POINT('Ctrl Pts',(37.3079892413964,-5.6523152960574,0.943208655172099));
#26753=CARTESIAN_POINT('Ctrl Pts',(37.8606208203438,-5.41997338236277,-1.86068203981508));
#26754=CARTESIAN_POINT('Ctrl Pts',(38.4132523992911,-3.88114100434969,-4.2160410449643));
#26755=CARTESIAN_POINT('Ctrl Pts',(38.9658839782385,-1.40674625429844,-5.55511740772306));
#26756=CARTESIAN_POINT('Ctrl Pts',(39.5185155571859,1.40674646354598,-5.55511666690852));
#26757=CARTESIAN_POINT('Ctrl Pts',(40.0711471361332,3.88114025546219,-4.21604221461142));
#26758=CARTESIAN_POINT('Ctrl Pts',(40.6237787150806,5.41997510425126,-1.86067976428242));
#26759=CARTESIAN_POINT('Ctrl Pts',(41.1764102940279,5.65231160321522,0.943203956408585));
#26760=CARTESIAN_POINT('Ctrl Pts',(41.7290418729754,4.52214418469897,3.51972611893208));
#26761=CARTESIAN_POINT('Ctrl Pts',(42.2816734519227,2.30190265803137,5.24780945677143));
#26762=CARTESIAN_POINT('Ctrl Pts',(42.8343050308701,-0.473218273533045,
5.71089524334113));
#26763=CARTESIAN_POINT('Ctrl Pts',(43.3869366098174,-3.13426874886167,4.79735545609104));
#26764=CARTESIAN_POINT('Ctrl Pts',(43.9395681887648,-5.03979591868312,2.72740116002078));
#26765=CARTESIAN_POINT('Ctrl Pts',(44.4921997677122,-5.73046769283071,-2.96113953592807E-10));
#26766=CARTESIAN_POINT('Ctrl Pts',(45.0448313466595,-5.03979591830015,-2.72740115925713));
#26767=CARTESIAN_POINT('Ctrl Pts',(45.5974629256069,-3.13426874984933,-4.79735545746814));
#26768=CARTESIAN_POINT('Ctrl Pts',(46.1500945045543,-0.473218271369011,
-5.71089524055342));
#26769=CARTESIAN_POINT('Ctrl Pts',(46.7027260835016,2.30190265343826,-5.24780946258346));
#26770=CARTESIAN_POINT('Ctrl Pts',(47.255357662449,4.52214419437993,-3.51972610673135));
#26771=CARTESIAN_POINT('Ctrl Pts',(47.8079892413964,5.65231158284243,-0.943203982060589));
#26772=CARTESIAN_POINT('Ctrl Pts',(48.3606208203438,5.41997514710894,1.86067981823473));
#26773=CARTESIAN_POINT('Ctrl Pts',(48.9132523992911,3.88114016531086,4.21604210112774));
#26774=CARTESIAN_POINT('Ctrl Pts',(49.4658839782385,1.40674665317661,5.55511690561523));
#26775=CARTESIAN_POINT('Ctrl Pts',(50.0185155571858,-1.40674665317677,5.5551169056147));
#26776=CARTESIAN_POINT('Ctrl Pts',(50.5711471361332,-3.8811401653103,4.2160421011286));
#26777=CARTESIAN_POINT('Ctrl Pts',(51.1237787150806,-5.4199751471102,1.86067981823306));
#26778=CARTESIAN_POINT('Ctrl Pts',(51.676410294028,-5.65231158283973,-0.943203982057156));
#26779=CARTESIAN_POINT('Ctrl Pts',(52.2290418729753,-4.52214419438563,-3.51972610673855));
#26780=CARTESIAN_POINT('Ctrl Pts',(52.7816734519227,-2.30190265342625,-5.24780946256834));
#26781=CARTESIAN_POINT('Ctrl Pts',(53.3343050308701,0.473218271343736,-5.71089524058523));
#26782=CARTESIAN_POINT('Ctrl Pts',(53.8869366098175,3.13426874990249,-4.79735545740122));
#26783=CARTESIAN_POINT('Ctrl Pts',(54.4395681887648,5.0397959181883,-2.72740115939791));
#26784=CARTESIAN_POINT('Ctrl Pts',(54.9921997677122,5.73046769306595,-5.11805824213355E-15));
#26785=CARTESIAN_POINT('Ctrl Pts',(55.5448313466596,5.03979591818831,2.72740115939791));
#26786=CARTESIAN_POINT('Ctrl Pts',(56.0974629256069,3.13426874990249,4.79735545740121));
#26787=CARTESIAN_POINT('Ctrl Pts',(56.6500945045543,0.473218271343732,5.71089524058523));
#26788=CARTESIAN_POINT('Ctrl Pts',(57.2027260835016,-2.30190265342626,5.24780946256833));
#26789=CARTESIAN_POINT('Ctrl Pts',(57.755357662449,-4.52214419438564,3.51972610673854));
#26790=CARTESIAN_POINT('Ctrl Pts',(58.3079892413963,-5.65231158283973,0.943203982057152));
#26791=CARTESIAN_POINT('Ctrl Pts',(58.8606208203438,-5.4199751471102,-1.86067981823306));
#26792=CARTESIAN_POINT('Ctrl Pts',(59.4132523992911,-3.88114016531031,-4.2160421011286));
#26793=CARTESIAN_POINT('Ctrl Pts',(59.9658839782385,-1.40674665317677,-5.55511690561469));
#26794=CARTESIAN_POINT('Ctrl Pts',(60.5185155571859,1.40674665317661,-5.55511690561524));
#26795=CARTESIAN_POINT('Ctrl Pts',(61.0711471361332,3.88114016531085,-4.21604210112775));
#26796=CARTESIAN_POINT('Ctrl Pts',(61.6237787150807,5.41997514710894,-1.86067981823474));
#26797=CARTESIAN_POINT('Ctrl Pts',(62.1764102940279,5.65231158284244,0.943203982060585));
#26798=CARTESIAN_POINT('Ctrl Pts',(62.7290418729753,4.52214419437993,3.51972610673135));
#26799=CARTESIAN_POINT('Ctrl Pts',(63.2816734519227,2.30190265343826,5.24780946258346));
#26800=CARTESIAN_POINT('Ctrl Pts',(63.8343050308701,-0.473218271369009,
5.71089524055341));
#26801=CARTESIAN_POINT('Ctrl Pts',(64.3869366098174,-3.13426874984932,4.79735545746814));
#26802=CARTESIAN_POINT('Ctrl Pts',(64.9395681887648,-5.03979591830014,2.72740115925714));
#26803=CARTESIAN_POINT('Ctrl Pts',(65.4921997677122,-5.73046769283071,2.96121409977839E-10));
#26804=CARTESIAN_POINT('Ctrl Pts',(66.0448313466595,-5.03979591868312,-2.72740116002078));
#26805=CARTESIAN_POINT('Ctrl Pts',(66.5974629256069,-3.13426874886167,-4.79735545609105));
#26806=CARTESIAN_POINT('Ctrl Pts',(67.1500945045543,-0.473218273533038,
-5.71089524334112));
#26807=CARTESIAN_POINT('Ctrl Pts',(67.7027260835016,2.30190265803138,-5.24780945677143));
#26808=CARTESIAN_POINT('Ctrl Pts',(68.255357662449,4.52214418469897,-3.51972611893208));
#26809=CARTESIAN_POINT('Ctrl Pts',(68.8079892413964,5.65231160321522,-0.943203956408587));
#26810=CARTESIAN_POINT('Ctrl Pts',(69.3606208203438,5.41997510425126,1.86067976428242));
#26811=CARTESIAN_POINT('Ctrl Pts',(69.9132523992911,3.88114025546219,4.21604221461142));
#26812=CARTESIAN_POINT('Ctrl Pts',(70.4658839782385,1.40674646354597,5.55511666690853));
#26813=CARTESIAN_POINT('Ctrl Pts',(71.0185155571859,-1.40674625429845,5.55511740772306));
#26814=CARTESIAN_POINT('Ctrl Pts',(71.5711471361332,-3.8811410043497,4.21604104496428));
#26815=CARTESIAN_POINT('Ctrl Pts',(72.1237787150806,-5.41997338236277,1.86068203981508));
#26816=CARTESIAN_POINT('Ctrl Pts',(72.676410294028,-5.65231529605741,-0.943208655172103));
#26817=CARTESIAN_POINT('Ctrl Pts',(73.2290418729754,-4.52213639346892,-3.51971627798694));
#26818=CARTESIAN_POINT('Ctrl Pts',(73.7816734519227,-2.30191914515453,-5.24783014539695));
#26819=CARTESIAN_POINT('Ctrl Pts',(74.3343050308701,0.473252278446422,-5.71085179682633));
#26820=CARTESIAN_POINT('Ctrl Pts',(74.8869366098175,3.13419106663809,-4.79744756259312));
#26821=CARTESIAN_POINT('Ctrl Pts',(75.4395681887648,5.03991467318512,-2.72720954086847));
#26822=CARTESIAN_POINT('Ctrl Pts',(75.8079892413964,5.49976642738082,-0.909403588662883));
#26823=CARTESIAN_POINT('Ctrl Pts',(75.9921997677122,5.49976642738082,-8.08232562162E-15));
#26824=CARTESIAN_POINT('',(75.9921997677122,5.49976642738082,-8.08232562162E-15));
#26825=CARTESIAN_POINT('',(33.9921997677122,5.49976642738082,0.));
#26826=CARTESIAN_POINT('Ctrl Pts',(75.9921997677122,5.49976642738082,-8.08232562162E-15));
#26827=CARTESIAN_POINT('Ctrl Pts',(75.8079892413964,5.49976642738082,-0.909403588662883));
#26828=CARTESIAN_POINT('Ctrl Pts',(75.4395681887648,5.03991467318512,-2.72720954086847));
#26829=CARTESIAN_POINT('Ctrl Pts',(74.8869366098175,3.13419106663809,-4.79744756259312));
#26830=CARTESIAN_POINT('Ctrl Pts',(74.3343050308701,0.473252278446422,-5.71085179682633));
#26831=CARTESIAN_POINT('Ctrl Pts',(73.7816734519227,-2.30191914515453,-5.24783014539695));
#26832=CARTESIAN_POINT('Ctrl Pts',(73.2290418729754,-4.52213639346892,-3.51971627798694));
#26833=CARTESIAN_POINT('Ctrl Pts',(72.676410294028,-5.65231529605741,-0.943208655172103));
#26834=CARTESIAN_POINT('Ctrl Pts',(72.1237787150806,-5.41997338236277,1.86068203981508));
#26835=CARTESIAN_POINT('Ctrl Pts',(71.5711471361332,-3.8811410043497,4.21604104496428));
#26836=CARTESIAN_POINT('Ctrl Pts',(71.0185155571859,-1.40674625429845,5.55511740772306));
#26837=CARTESIAN_POINT('Ctrl Pts',(70.4658839782385,1.40674646354597,5.55511666690853));
#26838=CARTESIAN_POINT('Ctrl Pts',(69.9132523992911,3.88114025546219,4.21604221461142));
#26839=CARTESIAN_POINT('Ctrl Pts',(69.3606208203438,5.41997510425126,1.86067976428242));
#26840=CARTESIAN_POINT('Ctrl Pts',(68.8079892413964,5.65231160321522,-0.943203956408587));
#26841=CARTESIAN_POINT('Ctrl Pts',(68.255357662449,4.52214418469897,-3.51972611893208));
#26842=CARTESIAN_POINT('Ctrl Pts',(67.7027260835016,2.30190265803138,-5.24780945677143));
#26843=CARTESIAN_POINT('Ctrl Pts',(67.1500945045543,-0.473218273533038,
-5.71089524334112));
#26844=CARTESIAN_POINT('Ctrl Pts',(66.5974629256069,-3.13426874886167,-4.79735545609105));
#26845=CARTESIAN_POINT('Ctrl Pts',(66.0448313466595,-5.03979591868312,-2.72740116002078));
#26846=CARTESIAN_POINT('Ctrl Pts',(65.4921997677122,-5.73046769283071,2.96121409977839E-10));
#26847=CARTESIAN_POINT('Ctrl Pts',(64.9395681887648,-5.03979591830014,2.72740115925714));
#26848=CARTESIAN_POINT('Ctrl Pts',(64.3869366098174,-3.13426874984932,4.79735545746814));
#26849=CARTESIAN_POINT('Ctrl Pts',(63.8343050308701,-0.473218271369009,
5.71089524055341));
#26850=CARTESIAN_POINT('Ctrl Pts',(63.2816734519227,2.30190265343826,5.24780946258346));
#26851=CARTESIAN_POINT('Ctrl Pts',(62.7290418729753,4.52214419437993,3.51972610673135));
#26852=CARTESIAN_POINT('Ctrl Pts',(62.1764102940279,5.65231158284244,0.943203982060585));
#26853=CARTESIAN_POINT('Ctrl Pts',(61.6237787150807,5.41997514710894,-1.86067981823474));
#26854=CARTESIAN_POINT('Ctrl Pts',(61.0711471361332,3.88114016531085,-4.21604210112775));
#26855=CARTESIAN_POINT('Ctrl Pts',(60.5185155571859,1.40674665317661,-5.55511690561524));
#26856=CARTESIAN_POINT('Ctrl Pts',(59.9658839782385,-1.40674665317677,-5.55511690561469));
#26857=CARTESIAN_POINT('Ctrl Pts',(59.4132523992911,-3.88114016531031,-4.2160421011286));
#26858=CARTESIAN_POINT('Ctrl Pts',(58.8606208203438,-5.4199751471102,-1.86067981823306));
#26859=CARTESIAN_POINT('Ctrl Pts',(58.3079892413963,-5.65231158283973,0.943203982057152));
#26860=CARTESIAN_POINT('Ctrl Pts',(57.755357662449,-4.52214419438564,3.51972610673854));
#26861=CARTESIAN_POINT('Ctrl Pts',(57.2027260835016,-2.30190265342626,5.24780946256833));
#26862=CARTESIAN_POINT('Ctrl Pts',(56.6500945045543,0.473218271343732,5.71089524058523));
#26863=CARTESIAN_POINT('Ctrl Pts',(56.0974629256069,3.13426874990249,4.79735545740121));
#26864=CARTESIAN_POINT('Ctrl Pts',(55.5448313466596,5.03979591818831,2.72740115939791));
#26865=CARTESIAN_POINT('Ctrl Pts',(54.9921997677122,5.73046769306595,-5.11805824213355E-15));
#26866=CARTESIAN_POINT('Ctrl Pts',(54.4395681887648,5.0397959181883,-2.72740115939791));
#26867=CARTESIAN_POINT('Ctrl Pts',(53.8869366098175,3.13426874990249,-4.79735545740122));
#26868=CARTESIAN_POINT('Ctrl Pts',(53.3343050308701,0.473218271343736,-5.71089524058523));
#26869=CARTESIAN_POINT('Ctrl Pts',(52.7816734519227,-2.30190265342625,-5.24780946256834));
#26870=CARTESIAN_POINT('Ctrl Pts',(52.2290418729753,-4.52214419438563,-3.51972610673855));
#26871=CARTESIAN_POINT('Ctrl Pts',(51.676410294028,-5.65231158283973,-0.943203982057156));
#26872=CARTESIAN_POINT('Ctrl Pts',(51.1237787150806,-5.4199751471102,1.86067981823306));
#26873=CARTESIAN_POINT('Ctrl Pts',(50.5711471361332,-3.8811401653103,4.2160421011286));
#26874=CARTESIAN_POINT('Ctrl Pts',(50.0185155571858,-1.40674665317677,5.5551169056147));
#26875=CARTESIAN_POINT('Ctrl Pts',(49.4658839782385,1.40674665317661,5.55511690561523));
#26876=CARTESIAN_POINT('Ctrl Pts',(48.9132523992911,3.88114016531086,4.21604210112774));
#26877=CARTESIAN_POINT('Ctrl Pts',(48.3606208203438,5.41997514710894,1.86067981823473));
#26878=CARTESIAN_POINT('Ctrl Pts',(47.8079892413964,5.65231158284243,-0.943203982060589));
#26879=CARTESIAN_POINT('Ctrl Pts',(47.255357662449,4.52214419437993,-3.51972610673135));
#26880=CARTESIAN_POINT('Ctrl Pts',(46.7027260835016,2.30190265343826,-5.24780946258346));
#26881=CARTESIAN_POINT('Ctrl Pts',(46.1500945045543,-0.473218271369011,
-5.71089524055342));
#26882=CARTESIAN_POINT('Ctrl Pts',(45.5974629256069,-3.13426874984933,-4.79735545746814));
#26883=CARTESIAN_POINT('Ctrl Pts',(45.0448313466595,-5.03979591830015,-2.72740115925713));
#26884=CARTESIAN_POINT('Ctrl Pts',(44.4921997677122,-5.73046769283071,-2.96113953592807E-10));
#26885=CARTESIAN_POINT('Ctrl Pts',(43.9395681887648,-5.03979591868312,2.72740116002078));
#26886=CARTESIAN_POINT('Ctrl Pts',(43.3869366098174,-3.13426874886167,4.79735545609104));
#26887=CARTESIAN_POINT('Ctrl Pts',(42.8343050308701,-0.473218273533045,
5.71089524334113));
#26888=CARTESIAN_POINT('Ctrl Pts',(42.2816734519227,2.30190265803137,5.24780945677143));
#26889=CARTESIAN_POINT('Ctrl Pts',(41.7290418729754,4.52214418469897,3.51972611893208));
#26890=CARTESIAN_POINT('Ctrl Pts',(41.1764102940279,5.65231160321522,0.943203956408585));
#26891=CARTESIAN_POINT('Ctrl Pts',(40.6237787150806,5.41997510425126,-1.86067976428242));
#26892=CARTESIAN_POINT('Ctrl Pts',(40.0711471361332,3.88114025546219,-4.21604221461142));
#26893=CARTESIAN_POINT('Ctrl Pts',(39.5185155571859,1.40674646354598,-5.55511666690852));
#26894=CARTESIAN_POINT('Ctrl Pts',(38.9658839782385,-1.40674625429844,-5.55511740772306));
#26895=CARTESIAN_POINT('Ctrl Pts',(38.4132523992911,-3.88114100434969,-4.2160410449643));
#26896=CARTESIAN_POINT('Ctrl Pts',(37.8606208203438,-5.41997338236277,-1.86068203981508));
#26897=CARTESIAN_POINT('Ctrl Pts',(37.3079892413964,-5.6523152960574,0.943208655172099));
#26898=CARTESIAN_POINT('Ctrl Pts',(36.755357662449,-4.52213639346893,3.51971627798693));
#26899=CARTESIAN_POINT('Ctrl Pts',(36.2027260835017,-2.30191914515453,5.24783014539696));
#26900=CARTESIAN_POINT('Ctrl Pts',(35.6500945045543,0.473252278446431,5.71085179682633));
#26901=CARTESIAN_POINT('Ctrl Pts',(35.0974629256069,3.13419106663809,4.79744756259311));
#26902=CARTESIAN_POINT('Ctrl Pts',(34.5448313466596,5.03991467318512,2.72720954086847));
#26903=CARTESIAN_POINT('Ctrl Pts',(34.176410294028,5.49976642738082,0.909403588662882));
#26904=CARTESIAN_POINT('Ctrl Pts',(33.9921997677122,5.49976642738082,0.));
#26905=CARTESIAN_POINT('',(74.9926516271063,5.5,-8.08266887437253E-15));
#26906=CARTESIAN_POINT('Ctrl Pts',(74.9926516271063,5.5,-8.88178419700125E-15));
#26907=CARTESIAN_POINT('Ctrl Pts',(74.9926516271063,5.49313135100536,-8.87169019419435E-15));
#26908=CARTESIAN_POINT('Ctrl Pts',(74.9928025594595,5.48616354876223,-8.85985100982881E-15));
#26909=CARTESIAN_POINT('Ctrl Pts',(74.9960623922239,5.41251939146685,-8.75162531201958E-15));
#26910=CARTESIAN_POINT('Ctrl Pts',(75.0129635856193,5.34674686927241,-8.64028104022342E-15));
#26911=CARTESIAN_POINT('Ctrl Pts',(75.0678279227212,5.23017858324776,-8.46897506618881E-15));
#26912=CARTESIAN_POINT('Ctrl Pts',(75.1045557576696,5.1784716444728,-8.3816878020062E-15));
#26913=CARTESIAN_POINT('Ctrl Pts',(75.2023392282651,5.08536492110004,-8.24486038109713E-15));
#26914=CARTESIAN_POINT('Ctrl Pts',(75.2593199555039,5.05418571732405,-7.68501720917694E-15));
#26915=CARTESIAN_POINT('Ctrl Pts',(75.3723346478213,5.01099405108005,-7.62154376619828E-15));
#26916=CARTESIAN_POINT('Ctrl Pts',(75.4380011585399,4.9992994690211,-7.59988681703217E-15));
#26917=CARTESIAN_POINT('Ctrl Pts',(75.5679318704974,5.00124746390966,-7.6027495438782E-15));
#26918=CARTESIAN_POINT('Ctrl Pts',(75.6303803662932,5.01468983699985,-7.77794865724713E-15));
#26919=CARTESIAN_POINT('Ctrl Pts',(75.7510076677018,5.06728521602235,-7.85524157233096E-15));
#26920=CARTESIAN_POINT('Ctrl Pts',(75.8069852154638,5.1062890809302,-7.92468346949603E-15));
#26921=CARTESIAN_POINT('Ctrl Pts',(75.8898187552,5.19148126768943,-8.0498798760885E-15));
#26922=CARTESIAN_POINT('Ctrl Pts',(75.9275855766847,5.24142762980879,-8.26790514855932E-15));
#26923=CARTESIAN_POINT('Ctrl Pts',(75.9798876154733,5.36745993607387,-8.45311922110734E-15));
#26924=CARTESIAN_POINT('Ctrl Pts',(75.992313334028,5.43375746391126,-8.78477899800761E-15));
#26925=CARTESIAN_POINT('Ctrl Pts',(75.9921997677122,5.49976642738082,-8.88178419700125E-15));
#26926=CARTESIAN_POINT('',(32.9926516271063,5.5,0.));
#26927=CARTESIAN_POINT('Ctrl Pts',(32.9926516271063,5.5,0.));
#26928=CARTESIAN_POINT('Ctrl Pts',(33.1768621534221,5.5,0.90940874905597));
#26929=CARTESIAN_POINT('Ctrl Pts',(33.5452832060536,5.0401165414414,2.72733561841164));
#26930=CARTESIAN_POINT('Ctrl Pts',(34.097914785001,3.13431992024721,4.79763437071315));
#26931=CARTESIAN_POINT('Ctrl Pts',(34.6505463639483,0.47327073373995,5.71108710593625));
#26932=CARTESIAN_POINT('Ctrl Pts',(35.2031779428958,-2.3020121722956,5.24804131697886));
#26933=CARTESIAN_POINT('Ctrl Pts',(35.7558095218431,-4.52232002588597,3.51985989359966));
#26934=CARTESIAN_POINT('Ctrl Pts',(36.3084411007905,-5.65254452743844,0.943246530010384));
#26935=CARTESIAN_POINT('Ctrl Pts',(36.8610726797378,-5.42019330761579,-1.86075734131042));
#26936=CARTESIAN_POINT('Ctrl Pts',(37.4137042586852,-3.88129844265893,-4.21621217675881));
#26937=CARTESIAN_POINT('Ctrl Pts',(37.9663358376326,-1.40680333428488,-5.55534273510501));
#26938=CARTESIAN_POINT('Ctrl Pts',(38.5189674165799,1.40680353896056,-5.55534205621606));
#26939=CARTESIAN_POINT('Ctrl Pts',(39.0715989955273,3.88129771013392,-4.21621324863341));
#26940=CARTESIAN_POINT('Ctrl Pts',(39.6242305744747,5.42019499188262,-1.86075525598994));
#26941=CARTESIAN_POINT('Ctrl Pts',(40.1768621534221,5.65254091528142,0.943242224042852));
#26942=CARTESIAN_POINT('Ctrl Pts',(40.7294937323694,4.52232764688486,3.51986891209907));
#26943=CARTESIAN_POINT('Ctrl Pts',(41.2821253113168,2.30199604540077,5.24802235924301));
#26944=CARTESIAN_POINT('Ctrl Pts',(41.8347568902642,-0.47323747180233,5.7111269323428));
#26945=CARTESIAN_POINT('Ctrl Pts',(42.3873884692115,-3.13439590518638,4.79755008340959));
#26946=CARTESIAN_POINT('Ctrl Pts',(42.9400200481589,-5.04000038161494,2.7275118097799));
#26947=CARTESIAN_POINT('Ctrl Pts',(43.4926516271062,-5.73070017611617,-2.71361235965901E-10));
#26948=CARTESIAN_POINT('Ctrl Pts',(44.0452832060537,-5.04000038124033,-2.72751180908009));
#26949=CARTESIAN_POINT('Ctrl Pts',(44.597914785001,-3.13439590615245,-4.79755008467159));
#26950=CARTESIAN_POINT('Ctrl Pts',(45.1505463639484,-0.473237469685579,
-5.71112692978812));
#26951=CARTESIAN_POINT('Ctrl Pts',(45.7031779428957,2.30199604090801,-5.2480223645692));
#26952=CARTESIAN_POINT('Ctrl Pts',(46.2558095218431,4.52232765635431,-3.5198689009182));
#26953=CARTESIAN_POINT('Ctrl Pts',(46.8084411007904,5.65254089535377,-0.943242247550575));
#26954=CARTESIAN_POINT('Ctrl Pts',(47.3610726797379,5.4201950338039,1.86075530543231));
#26955=CARTESIAN_POINT('Ctrl Pts',(47.9137042586852,3.88129762195231,4.21621314463597));
#26956=CARTESIAN_POINT('Ctrl Pts',(48.4663358376326,1.40680372444794,5.55534227496898));
#26957=CARTESIAN_POINT('Ctrl Pts',(49.0189674165799,-1.40680372444809,5.55534227496848));
#26958=CARTESIAN_POINT('Ctrl Pts',(49.5715989955273,-3.88129762195177,4.21621314463675));
#26959=CARTESIAN_POINT('Ctrl Pts',(50.1242305744747,-5.42019503380513,1.86075530543079));
#26960=CARTESIAN_POINT('Ctrl Pts',(50.6768621534221,-5.65254089535113,-0.943242247547429));
#26961=CARTESIAN_POINT('Ctrl Pts',(51.2294937323694,-4.52232765635988,-3.51986890092481));
#26962=CARTESIAN_POINT('Ctrl Pts',(51.7821253113168,-2.30199604089626,-5.24802236455534));
#26963=CARTESIAN_POINT('Ctrl Pts',(52.3347568902641,0.473237469660857,-5.71112692981728));
#26964=CARTESIAN_POINT('Ctrl Pts',(52.8873884692115,3.13439590620446,-4.79755008461025));
#26965=CARTESIAN_POINT('Ctrl Pts',(53.4400200481589,5.04000038113094,-2.7275118092091));
#26966=CARTESIAN_POINT('Ctrl Pts',(53.9926516271062,5.73070017634626,-5.09570864282292E-15));
#26967=CARTESIAN_POINT('Ctrl Pts',(54.5452832060537,5.04000038113094,2.7275118092091));
#26968=CARTESIAN_POINT('Ctrl Pts',(55.0979147850009,3.13439590620446,4.79755008461025));
#26969=CARTESIAN_POINT('Ctrl Pts',(55.6505463639484,0.473237469660853,5.71112692981727));
#26970=CARTESIAN_POINT('Ctrl Pts',(56.2031779428957,-2.30199604089627,5.24802236455534));
#26971=CARTESIAN_POINT('Ctrl Pts',(56.7558095218432,-4.52232765635989,3.5198689009248));
#26972=CARTESIAN_POINT('Ctrl Pts',(57.3084411007904,-5.65254089535113,0.943242247547423));
#26973=CARTESIAN_POINT('Ctrl Pts',(57.8610726797378,-5.42019503380513,-1.86075530543079));
#26974=CARTESIAN_POINT('Ctrl Pts',(58.4137042586852,-3.88129762195177,-4.21621314463675));
#26975=CARTESIAN_POINT('Ctrl Pts',(58.9663358376325,-1.4068037244481,-5.55534227496848));
#26976=CARTESIAN_POINT('Ctrl Pts',(59.51896741658,1.40680372444794,-5.55534227496898));
#26977=CARTESIAN_POINT('Ctrl Pts',(60.0715989955273,3.88129762195231,-4.21621314463597));
#26978=CARTESIAN_POINT('Ctrl Pts',(60.6242305744747,5.4201950338039,-1.86075530543232));
#26979=CARTESIAN_POINT('Ctrl Pts',(61.176862153422,5.65254089535377,0.94324224755057));
#26980=CARTESIAN_POINT('Ctrl Pts',(61.7294937323694,4.52232765635431,3.5198689009182));
#26981=CARTESIAN_POINT('Ctrl Pts',(62.2821253113167,2.30199604090801,5.2480223645692));
#26982=CARTESIAN_POINT('Ctrl Pts',(62.8347568902642,-0.473237469685578,
5.71112692978812));
#26983=CARTESIAN_POINT('Ctrl Pts',(63.3873884692115,-3.13439590615245,4.79755008467159));
#26984=CARTESIAN_POINT('Ctrl Pts',(63.9400200481589,-5.04000038124033,2.7275118090801));
#26985=CARTESIAN_POINT('Ctrl Pts',(64.4926516271063,-5.73070017611617,2.71368745431234E-10));
#26986=CARTESIAN_POINT('Ctrl Pts',(65.0452832060536,-5.04000038161494,-2.7275118097799));
#26987=CARTESIAN_POINT('Ctrl Pts',(65.597914785001,-3.13439590518638,-4.7975500834096));
#26988=CARTESIAN_POINT('Ctrl Pts',(66.1505463639483,-0.473237471802323,
-5.7111269323428));
#26989=CARTESIAN_POINT('Ctrl Pts',(66.7031779428957,2.30199604540077,-5.248022359243));
#26990=CARTESIAN_POINT('Ctrl Pts',(67.255809521843,4.52232764688486,-3.51986891209906));
#26991=CARTESIAN_POINT('Ctrl Pts',(67.8084411007905,5.65254091528143,-0.943242224042853));
#26992=CARTESIAN_POINT('Ctrl Pts',(68.3610726797379,5.42019499188262,1.86075525598994));
#26993=CARTESIAN_POINT('Ctrl Pts',(68.9137042586851,3.88129771013392,4.21621324863341));
#26994=CARTESIAN_POINT('Ctrl Pts',(69.4663358376326,1.40680353896055,5.55534205621606));
#26995=CARTESIAN_POINT('Ctrl Pts',(70.0189674165799,-1.4068033342849,5.55534273510501));
#26996=CARTESIAN_POINT('Ctrl Pts',(70.5715989955273,-3.88129844265893,4.21621217675881));
#26997=CARTESIAN_POINT('Ctrl Pts',(71.1242305744747,-5.42019330761579,1.86075734131042));
#26998=CARTESIAN_POINT('Ctrl Pts',(71.6768621534221,-5.65254452743844,-0.943246530010386));
#26999=CARTESIAN_POINT('Ctrl Pts',(72.2294937323694,-4.52232002588597,-3.51985989359967));
#27000=CARTESIAN_POINT('Ctrl Pts',(72.7821253113168,-2.3020121722956,-5.24804131697885));
#27001=CARTESIAN_POINT('Ctrl Pts',(73.3347568902641,0.47327073373994,-5.71108710593626));
#27002=CARTESIAN_POINT('Ctrl Pts',(73.8873884692115,3.13431992024721,-4.79763437071315));
#27003=CARTESIAN_POINT('Ctrl Pts',(74.4400200481589,5.04011654144139,-2.72733561841164));
#27004=CARTESIAN_POINT('Ctrl Pts',(74.8084411007905,5.5,-0.909408749055971));
#27005=CARTESIAN_POINT('Ctrl Pts',(74.9926516271063,5.5,-8.08266887437253E-15));
#27006=CARTESIAN_POINT('Ctrl Pts',(32.9926516271063,5.5,-1.33481475863792E-22));
#27007=CARTESIAN_POINT('Ctrl Pts',(32.9926516271063,5.49313135093644,-1.33481475863792E-22));
#27008=CARTESIAN_POINT('Ctrl Pts',(32.9928025594625,5.48616354862232,0.));
#27009=CARTESIAN_POINT('Ctrl Pts',(32.9960623922631,5.41251939125576,0.));
#27010=CARTESIAN_POINT('Ctrl Pts',(33.012963585686,5.34674686906042,0.));
#27011=CARTESIAN_POINT('Ctrl Pts',(33.0678279228392,5.23017858306288,0.));
#27012=CARTESIAN_POINT('Ctrl Pts',(33.1045557578012,5.17847164431084,0.));
#27013=CARTESIAN_POINT('Ctrl Pts',(33.202339228433,5.08536492098311,0.));
#27014=CARTESIAN_POINT('Ctrl Pts',(33.2593199556946,5.054185717226,0.));
#27015=CARTESIAN_POINT('Ctrl Pts',(33.3723346480206,5.01099405103351,0.));
#27016=CARTESIAN_POINT('Ctrl Pts',(33.4380011587359,4.99929946899863,0.));
#27017=CARTESIAN_POINT('Ctrl Pts',(33.5679318706913,5.0012474639378,0.));
#27018=CARTESIAN_POINT('Ctrl Pts',(33.6303803664784,5.01468983705302,0.));
#27019=CARTESIAN_POINT('Ctrl Pts',(33.75100766786,5.06728521611982,0.));
#27020=CARTESIAN_POINT('Ctrl Pts',(33.8069852156061,5.10628908104261,0.));
#27021=CARTESIAN_POINT('Ctrl Pts',(33.8898187553161,5.19148126783547,0.));
#27022=CARTESIAN_POINT('Ctrl Pts',(33.9275855767874,5.24142762997304,0.));
#27023=CARTESIAN_POINT('Ctrl Pts',(33.9798876154972,5.36745993620988,0.));
#27024=CARTESIAN_POINT('Ctrl Pts',(33.9923133340279,5.4337574639749,5.17361254957654E-35));
#27025=CARTESIAN_POINT('Ctrl Pts',(33.9921997677122,5.49976642738082,5.17361254957654E-35));
#27026=CARTESIAN_POINT('Ctrl Pts',(33.9921997677122,5.49976642738082,0.));
#27027=CARTESIAN_POINT('Ctrl Pts',(34.176410294028,5.49976642738082,0.909403588662882));
#27028=CARTESIAN_POINT('Ctrl Pts',(34.5448313466596,5.03991467318512,2.72720954086847));
#27029=CARTESIAN_POINT('Ctrl Pts',(35.0974629256069,3.13419106663809,4.79744756259311));
#27030=CARTESIAN_POINT('Ctrl Pts',(35.6500945045543,0.473252278446431,5.71085179682633));
#27031=CARTESIAN_POINT('Ctrl Pts',(36.2027260835017,-2.30191914515453,5.24783014539696));
#27032=CARTESIAN_POINT('Ctrl Pts',(36.755357662449,-4.52213639346893,3.51971627798693));
#27033=CARTESIAN_POINT('Ctrl Pts',(37.3079892413964,-5.6523152960574,0.943208655172099));
#27034=CARTESIAN_POINT('Ctrl Pts',(37.8606208203438,-5.41997338236277,-1.86068203981508));
#27035=CARTESIAN_POINT('Ctrl Pts',(38.4132523992911,-3.88114100434969,-4.2160410449643));
#27036=CARTESIAN_POINT('Ctrl Pts',(38.9658839782385,-1.40674625429844,-5.55511740772306));
#27037=CARTESIAN_POINT('Ctrl Pts',(39.5185155571859,1.40674646354598,-5.55511666690852));
#27038=CARTESIAN_POINT('Ctrl Pts',(40.0711471361332,3.88114025546219,-4.21604221461142));
#27039=CARTESIAN_POINT('Ctrl Pts',(40.6237787150806,5.41997510425126,-1.86067976428242));
#27040=CARTESIAN_POINT('Ctrl Pts',(41.1764102940279,5.65231160321522,0.943203956408585));
#27041=CARTESIAN_POINT('Ctrl Pts',(41.7290418729754,4.52214418469897,3.51972611893208));
#27042=CARTESIAN_POINT('Ctrl Pts',(42.2816734519227,2.30190265803137,5.24780945677143));
#27043=CARTESIAN_POINT('Ctrl Pts',(42.8343050308701,-0.473218273533045,
5.71089524334113));
#27044=CARTESIAN_POINT('Ctrl Pts',(43.3869366098174,-3.13426874886167,4.79735545609104));
#27045=CARTESIAN_POINT('Ctrl Pts',(43.9395681887648,-5.03979591868312,2.72740116002078));
#27046=CARTESIAN_POINT('Ctrl Pts',(44.4921997677122,-5.73046769283071,-2.96113953592807E-10));
#27047=CARTESIAN_POINT('Ctrl Pts',(45.0448313466595,-5.03979591830015,-2.72740115925713));
#27048=CARTESIAN_POINT('Ctrl Pts',(45.5974629256069,-3.13426874984933,-4.79735545746814));
#27049=CARTESIAN_POINT('Ctrl Pts',(46.1500945045543,-0.473218271369011,
-5.71089524055342));
#27050=CARTESIAN_POINT('Ctrl Pts',(46.7027260835016,2.30190265343826,-5.24780946258346));
#27051=CARTESIAN_POINT('Ctrl Pts',(47.255357662449,4.52214419437993,-3.51972610673135));
#27052=CARTESIAN_POINT('Ctrl Pts',(47.8079892413964,5.65231158284243,-0.943203982060589));
#27053=CARTESIAN_POINT('Ctrl Pts',(48.3606208203438,5.41997514710894,1.86067981823473));
#27054=CARTESIAN_POINT('Ctrl Pts',(48.9132523992911,3.88114016531086,4.21604210112774));
#27055=CARTESIAN_POINT('Ctrl Pts',(49.4658839782385,1.40674665317661,5.55511690561523));
#27056=CARTESIAN_POINT('Ctrl Pts',(50.0185155571858,-1.40674665317677,5.5551169056147));
#27057=CARTESIAN_POINT('Ctrl Pts',(50.5711471361332,-3.8811401653103,4.2160421011286));
#27058=CARTESIAN_POINT('Ctrl Pts',(51.1237787150806,-5.4199751471102,1.86067981823306));
#27059=CARTESIAN_POINT('Ctrl Pts',(51.676410294028,-5.65231158283973,-0.943203982057156));
#27060=CARTESIAN_POINT('Ctrl Pts',(52.2290418729753,-4.52214419438563,-3.51972610673855));
#27061=CARTESIAN_POINT('Ctrl Pts',(52.7816734519227,-2.30190265342625,-5.24780946256834));
#27062=CARTESIAN_POINT('Ctrl Pts',(53.3343050308701,0.473218271343736,-5.71089524058523));
#27063=CARTESIAN_POINT('Ctrl Pts',(53.8869366098175,3.13426874990249,-4.79735545740122));
#27064=CARTESIAN_POINT('Ctrl Pts',(54.4395681887648,5.0397959181883,-2.72740115939791));
#27065=CARTESIAN_POINT('Ctrl Pts',(54.9921997677122,5.73046769306595,-5.11805824213355E-15));
#27066=CARTESIAN_POINT('Ctrl Pts',(55.5448313466596,5.03979591818831,2.72740115939791));
#27067=CARTESIAN_POINT('Ctrl Pts',(56.0974629256069,3.13426874990249,4.79735545740121));
#27068=CARTESIAN_POINT('Ctrl Pts',(56.6500945045543,0.473218271343732,5.71089524058523));
#27069=CARTESIAN_POINT('Ctrl Pts',(57.2027260835016,-2.30190265342626,5.24780946256833));
#27070=CARTESIAN_POINT('Ctrl Pts',(57.755357662449,-4.52214419438564,3.51972610673854));
#27071=CARTESIAN_POINT('Ctrl Pts',(58.3079892413963,-5.65231158283973,0.943203982057152));
#27072=CARTESIAN_POINT('Ctrl Pts',(58.8606208203438,-5.4199751471102,-1.86067981823306));
#27073=CARTESIAN_POINT('Ctrl Pts',(59.4132523992911,-3.88114016531031,-4.2160421011286));
#27074=CARTESIAN_POINT('Ctrl Pts',(59.9658839782385,-1.40674665317677,-5.55511690561469));
#27075=CARTESIAN_POINT('Ctrl Pts',(60.5185155571859,1.40674665317661,-5.55511690561524));
#27076=CARTESIAN_POINT('Ctrl Pts',(61.0711471361332,3.88114016531085,-4.21604210112775));
#27077=CARTESIAN_POINT('Ctrl Pts',(61.6237787150807,5.41997514710894,-1.86067981823474));
#27078=CARTESIAN_POINT('Ctrl Pts',(62.1764102940279,5.65231158284244,0.943203982060585));
#27079=CARTESIAN_POINT('Ctrl Pts',(62.7290418729753,4.52214419437993,3.51972610673135));
#27080=CARTESIAN_POINT('Ctrl Pts',(63.2816734519227,2.30190265343826,5.24780946258346));
#27081=CARTESIAN_POINT('Ctrl Pts',(63.8343050308701,-0.473218271369009,
5.71089524055341));
#27082=CARTESIAN_POINT('Ctrl Pts',(64.3869366098174,-3.13426874984932,4.79735545746814));
#27083=CARTESIAN_POINT('Ctrl Pts',(64.9395681887648,-5.03979591830014,2.72740115925714));
#27084=CARTESIAN_POINT('Ctrl Pts',(65.4921997677122,-5.73046769283071,2.96121409977839E-10));
#27085=CARTESIAN_POINT('Ctrl Pts',(66.0448313466595,-5.03979591868312,-2.72740116002078));
#27086=CARTESIAN_POINT('Ctrl Pts',(66.5974629256069,-3.13426874886167,-4.79735545609105));
#27087=CARTESIAN_POINT('Ctrl Pts',(67.1500945045543,-0.473218273533038,
-5.71089524334112));
#27088=CARTESIAN_POINT('Ctrl Pts',(67.7027260835016,2.30190265803138,-5.24780945677143));
#27089=CARTESIAN_POINT('Ctrl Pts',(68.255357662449,4.52214418469897,-3.51972611893208));
#27090=CARTESIAN_POINT('Ctrl Pts',(68.8079892413964,5.65231160321522,-0.943203956408587));
#27091=CARTESIAN_POINT('Ctrl Pts',(69.3606208203438,5.41997510425126,1.86067976428242));
#27092=CARTESIAN_POINT('Ctrl Pts',(69.9132523992911,3.88114025546219,4.21604221461142));
#27093=CARTESIAN_POINT('Ctrl Pts',(70.4658839782385,1.40674646354597,5.55511666690853));
#27094=CARTESIAN_POINT('Ctrl Pts',(71.0185155571859,-1.40674625429845,5.55511740772306));
#27095=CARTESIAN_POINT('Ctrl Pts',(71.5711471361332,-3.8811410043497,4.21604104496428));
#27096=CARTESIAN_POINT('Ctrl Pts',(72.1237787150806,-5.41997338236277,1.86068203981508));
#27097=CARTESIAN_POINT('Ctrl Pts',(72.676410294028,-5.65231529605741,-0.943208655172103));
#27098=CARTESIAN_POINT('Ctrl Pts',(73.2290418729754,-4.52213639346892,-3.51971627798694));
#27099=CARTESIAN_POINT('Ctrl Pts',(73.7816734519227,-2.30191914515453,-5.24783014539695));
#27100=CARTESIAN_POINT('Ctrl Pts',(74.3343050308701,0.473252278446422,-5.71085179682633));
#27101=CARTESIAN_POINT('Ctrl Pts',(74.8869366098175,3.13419106663809,-4.79744756259312));
#27102=CARTESIAN_POINT('Ctrl Pts',(75.4395681887648,5.03991467318512,-2.72720954086847));
#27103=CARTESIAN_POINT('Ctrl Pts',(75.8079892413964,5.49976642738082,-0.909403588662883));
#27104=CARTESIAN_POINT('Ctrl Pts',(75.9921997677122,5.49976642738082,-8.08232562162E-15));
#27105=CARTESIAN_POINT('Ctrl Pts',(33.9920707665653,5.57474668825,0.));
#27106=CARTESIAN_POINT('Ctrl Pts',(34.1762812928811,5.57474668825,0.921801519276635));
#27107=CARTESIAN_POINT('Ctrl Pts',(34.5447023455127,5.10862550688029,2.76439064201748));
#27108=CARTESIAN_POINT('Ctrl Pts',(35.0973339244601,3.17692056506673,4.86285271511581));
#27109=CARTESIAN_POINT('Ctrl Pts',(35.6499655034074,0.479704279887822,5.78870979651738));
#27110=CARTESIAN_POINT('Ctrl Pts',(36.2025970823548,-2.33330198195422,5.31937556836421));
#27111=CARTESIAN_POINT('Ctrl Pts',(36.7552286613021,-4.5837882052994,3.56770176400508));
#27112=CARTESIAN_POINT('Ctrl Pts',(37.3078602402495,-5.72937521578602,0.956067733435914));
#27113=CARTESIAN_POINT('Ctrl Pts',(37.8604918191969,-5.49386570747434,-1.88604934388851));
#27114=CARTESIAN_POINT('Ctrl Pts',(38.4131233981442,-3.93405390825201,-4.27351975497624));
#27115=CARTESIAN_POINT('Ctrl Pts',(38.9657549770916,-1.42592490042418,-5.63085219620485));
#27116=CARTESIAN_POINT('Ctrl Pts',(39.518386556039,1.42592511248475,-5.63085144582777));
#27117=CARTESIAN_POINT('Ctrl Pts',(40.0710181349864,3.93405314929682,-4.27352093972135));
#27118=CARTESIAN_POINT('Ctrl Pts',(40.6236497139337,5.4938674525111,-1.8860470389829));
#27119=CARTESIAN_POINT('Ctrl Pts',(41.176281292881,5.729371473299,0.95606297402021));
#27120=CARTESIAN_POINT('Ctrl Pts',(41.7289128718285,4.58379610127107,3.56771173198016));
#27121=CARTESIAN_POINT('Ctrl Pts',(42.2815444507758,2.33328527318593,5.31935461269972));
#27122=CARTESIAN_POINT('Ctrl Pts',(42.8341760297232,-0.479669817828385,
5.78875380394745));
#27123=CARTESIAN_POINT('Ctrl Pts',(43.3868076086705,-3.17699929161356,4.8627594207284));
#27124=CARTESIAN_POINT('Ctrl Pts',(43.9394391876179,-5.10850515589866,2.76458473973461));
#27125=CARTESIAN_POINT('Ctrl Pts',(44.4920707665653,-5.80859309124294,-2.99936115018113E-10));
#27126=CARTESIAN_POINT('Ctrl Pts',(45.0447023455126,-5.10850515551054,-2.7645847389611));
#27127=CARTESIAN_POINT('Ctrl Pts',(45.59733392446,-3.17699929261449,-4.86275942212328));
#27128=CARTESIAN_POINT('Ctrl Pts',(46.1499655034074,-0.479669815635259,
-5.78875380112376));
#27129=CARTESIAN_POINT('Ctrl Pts',(46.7025970823548,2.33328526853108,-5.31935461858677));
#27130=CARTESIAN_POINT('Ctrl Pts',(47.2552286613021,4.58379611108217,-3.56771171962194));
#27131=CARTESIAN_POINT('Ctrl Pts',(47.8078602402495,5.72937145265234,-0.956063000003334));
#27132=CARTESIAN_POINT('Ctrl Pts',(48.3604918191969,5.49386749594493,1.88604709363163));
#27133=CARTESIAN_POINT('Ctrl Pts',(48.9131233981442,3.93405305793353,4.27352082477281));
#27134=CARTESIAN_POINT('Ctrl Pts',(49.4657549770916,1.42592530466468,5.63085168761574));
#27135=CARTESIAN_POINT('Ctrl Pts',(50.018386556039,-1.42592530466484,5.6308516876152));
#27136=CARTESIAN_POINT('Ctrl Pts',(50.5710181349864,-3.93405305793297,4.27352082477367));
#27137=CARTESIAN_POINT('Ctrl Pts',(51.1236497139337,-5.49386749594621,1.88604709362994));
#27138=CARTESIAN_POINT('Ctrl Pts',(51.6762812928811,-5.7293714526496,-0.956062999999857));
#27139=CARTESIAN_POINT('Ctrl Pts',(52.2289128718284,-4.58379611108795,-3.56771171962923));
#27140=CARTESIAN_POINT('Ctrl Pts',(52.7815444507759,-2.3332852685189,-5.31935461857145));
#27141=CARTESIAN_POINT('Ctrl Pts',(53.3341760297232,0.479669815609644,-5.78875380115598));
#27142=CARTESIAN_POINT('Ctrl Pts',(53.8868076086706,3.17699929266837,-4.86275942205549));
#27143=CARTESIAN_POINT('Ctrl Pts',(54.4394391876179,5.10850515539719,-2.7645847391037));
#27144=CARTESIAN_POINT('Ctrl Pts',(54.9920707665653,5.80859309148135,-5.41419043299935E-15));
#27145=CARTESIAN_POINT('Ctrl Pts',(55.5447023455127,5.1085051553972,2.7645847391037));
#27146=CARTESIAN_POINT('Ctrl Pts',(56.0973339244601,3.17699929266837,4.86275942205548));
#27147=CARTESIAN_POINT('Ctrl Pts',(56.6499655034074,0.47966981560964,5.78875380115598));
#27148=CARTESIAN_POINT('Ctrl Pts',(57.2025970823548,-2.33328526851891,5.31935461857144));
#27149=CARTESIAN_POINT('Ctrl Pts',(57.7552286613021,-4.58379611108796,3.56771171962922));
#27150=CARTESIAN_POINT('Ctrl Pts',(58.3078602402495,-5.7293714526496,0.956062999999852));
#27151=CARTESIAN_POINT('Ctrl Pts',(58.8604918191969,-5.49386749594621,-1.88604709362995));
#27152=CARTESIAN_POINT('Ctrl Pts',(59.4131233981442,-3.93405305793297,-4.27352082477368));
#27153=CARTESIAN_POINT('Ctrl Pts',(59.9657549770916,-1.42592530466484,-5.63085168761519));
#27154=CARTESIAN_POINT('Ctrl Pts',(60.518386556039,1.42592530466468,-5.63085168761575));
#27155=CARTESIAN_POINT('Ctrl Pts',(61.0710181349863,3.93405305793353,-4.27352082477281));
#27156=CARTESIAN_POINT('Ctrl Pts',(61.6236497139338,5.49386749594494,-1.88604709363164));
#27157=CARTESIAN_POINT('Ctrl Pts',(62.1762812928811,5.72937145265234,0.95606300000333));
#27158=CARTESIAN_POINT('Ctrl Pts',(62.7289128718285,4.58379611108217,3.56771171962194));
#27159=CARTESIAN_POINT('Ctrl Pts',(63.2815444507758,2.33328526853108,5.31935461858677));
#27160=CARTESIAN_POINT('Ctrl Pts',(63.8341760297232,-0.479669815635258,
5.78875380112375));
#27161=CARTESIAN_POINT('Ctrl Pts',(64.3868076086705,-3.17699929261449,4.86275942212328));
#27162=CARTESIAN_POINT('Ctrl Pts',(64.9394391876179,-5.10850515551053,2.76458473896111));
#27163=CARTESIAN_POINT('Ctrl Pts',(65.4920707665653,-5.80859309124295,2.9994369153224E-10));
#27164=CARTESIAN_POINT('Ctrl Pts',(66.0447023455127,-5.10850515589866,-2.76458473973461));
#27165=CARTESIAN_POINT('Ctrl Pts',(66.59733392446,-3.17699929161356,-4.86275942072841));
#27166=CARTESIAN_POINT('Ctrl Pts',(67.1499655034074,-0.479669817828379,
-5.78875380394745));
#27167=CARTESIAN_POINT('Ctrl Pts',(67.7025970823548,2.33328527318594,-5.31935461269972));
#27168=CARTESIAN_POINT('Ctrl Pts',(68.2552286613022,4.58379610127107,-3.56771173198016));
#27169=CARTESIAN_POINT('Ctrl Pts',(68.8078602402495,5.72937147329901,-0.956062974020212));
#27170=CARTESIAN_POINT('Ctrl Pts',(69.3604918191969,5.4938674525111,1.8860470389829));
#27171=CARTESIAN_POINT('Ctrl Pts',(69.9131233981443,3.93405314929682,4.27352093972134));
#27172=CARTESIAN_POINT('Ctrl Pts',(70.4657549770917,1.42592511248473,5.63085144582777));
#27173=CARTESIAN_POINT('Ctrl Pts',(71.018386556039,-1.42592490042419,5.63085219620485));
#27174=CARTESIAN_POINT('Ctrl Pts',(71.5710181349864,-3.93405390825202,4.27351975497623));
#27175=CARTESIAN_POINT('Ctrl Pts',(72.1236497139337,-5.49386570747434,1.88604934388851));
#27176=CARTESIAN_POINT('Ctrl Pts',(72.6762812928811,-5.72937521578603,-0.956067733435918));
#27177=CARTESIAN_POINT('Ctrl Pts',(73.2289128718285,-4.58378820529939,-3.56770176400509));
#27178=CARTESIAN_POINT('Ctrl Pts',(73.7815444507758,-2.33330198195422,-5.31937556836421));
#27179=CARTESIAN_POINT('Ctrl Pts',(74.3341760297232,0.479704279887813,-5.78870979651738));
#27180=CARTESIAN_POINT('Ctrl Pts',(74.8868076086706,3.17692056506672,-4.86285271511582));
#27181=CARTESIAN_POINT('Ctrl Pts',(75.4394391876179,5.10862550688029,-2.76439064201748));
#27182=CARTESIAN_POINT('Ctrl Pts',(75.8078602402495,5.57474668825,-0.921801519276636));
#27183=CARTESIAN_POINT('Ctrl Pts',(75.9920707665653,5.57474668825,-8.19251482538721E-15));
#27184=CARTESIAN_POINT('Ctrl Pts',(33.9431414536155,5.79981109503712,0.));
#27185=CARTESIAN_POINT('Ctrl Pts',(34.1273519799313,5.79981109503712,0.95899747143683));
#27186=CARTESIAN_POINT('Ctrl Pts',(34.4957730325629,5.31486464408031,2.87600085013837));
#27187=CARTESIAN_POINT('Ctrl Pts',(35.0484046115103,3.30517718677737,5.05916675657821));
#27188=CARTESIAN_POINT('Ctrl Pts',(35.6010361904576,0.499070024096898,6.02240821551781));
#27189=CARTESIAN_POINT('Ctrl Pts',(36.153667769405,-2.42749964852484,5.53412340547436));
#27190=CARTESIAN_POINT('Ctrl Pts',(36.7062993483523,-4.76884068918239,3.71173413415615));
#27191=CARTESIAN_POINT('Ctrl Pts',(37.2589309272997,-5.96067611682369,0.994664977192594));
#27192=CARTESIAN_POINT('Ctrl Pts',(37.8115625062471,-5.71565890873659,-1.96219104782992));
#27193=CARTESIAN_POINT('Ctrl Pts',(38.3641940851944,-4.09287582201278,-4.4460463256512));
#27194=CARTESIAN_POINT('Ctrl Pts',(38.9168256641418,-1.48349100436533,-5.85817564103365));
#27195=CARTESIAN_POINT('Ctrl Pts',(39.4694572430892,1.48349122236704,-5.85817489580175));
#27196=CARTESIAN_POINT('Ctrl Pts',(40.0220888220366,4.09287504179451,-4.44604750227257));
#27197=CARTESIAN_POINT('Ctrl Pts',(40.5747204009839,5.71566070266274,-1.96218875872725));
#27198=CARTESIAN_POINT('Ctrl Pts',(41.1273519799312,5.96067226948622,0.994660250423079));
#27199=CARTESIAN_POINT('Ctrl Pts',(41.6799835588787,4.76884880636957,3.71174403388056));
#27200=CARTESIAN_POINT('Ctrl Pts',(42.232615137826,2.42748247163953,5.5341025943587));
#27201=CARTESIAN_POINT('Ctrl Pts',(42.7852467167734,-0.499034596539813,
6.0224519278597));
#27202=CARTESIAN_POINT('Ctrl Pts',(43.3378782957207,-3.30525811894677,5.0590741705265));
#27203=CARTESIAN_POINT('Ctrl Pts',(43.8905098746681,-5.31474092131558,2.87619395462708));
#27204=CARTESIAN_POINT('Ctrl Pts',(44.4431414536155,-6.04309214833711,-2.97879057897562E-10));
#27205=CARTESIAN_POINT('Ctrl Pts',(44.9957730325628,-5.31474092091659,-2.87619395385888));
#27206=CARTESIAN_POINT('Ctrl Pts',(45.5484046115102,-3.30525811997574,-5.05907417191182));
#27207=CARTESIAN_POINT('Ctrl Pts',(46.1010361904576,-0.499034594285245,
-6.02245192505537));
#27208=CARTESIAN_POINT('Ctrl Pts',(46.653667769405,2.42748246685427,-5.53410260020539));
#27209=CARTESIAN_POINT('Ctrl Pts',(47.2062993483523,4.76884881645555,-3.71174402160707));
#27210=CARTESIAN_POINT('Ctrl Pts',(47.7589309272997,5.96067224826112,-0.994660276228043));
#27211=CARTESIAN_POINT('Ctrl Pts',(48.3115625062471,5.71566074731342,1.96218881300126));
#27212=CARTESIAN_POINT('Ctrl Pts',(48.8641940851944,4.09287494787157,4.44604738811221));
#27213=CARTESIAN_POINT('Ctrl Pts',(49.4168256641418,1.48349141993114,5.85817513593182));
#27214=CARTESIAN_POINT('Ctrl Pts',(49.9694572430891,-1.48349141993129,5.85817513593129));
#27215=CARTESIAN_POINT('Ctrl Pts',(50.5220888220366,-4.09287494787099,4.44604738811307));
#27216=CARTESIAN_POINT('Ctrl Pts',(51.0747204009839,-5.71566074731474,1.96218881299959));
#27217=CARTESIAN_POINT('Ctrl Pts',(51.6273519799313,-5.96067224825831,-0.994660276224589));
#27218=CARTESIAN_POINT('Ctrl Pts',(52.1799835588786,-4.76884881646149,-3.71174402161432));
#27219=CARTESIAN_POINT('Ctrl Pts',(52.7326151378261,-2.42748246684175,-5.53410260019018));
#27220=CARTESIAN_POINT('Ctrl Pts',(53.2852467167734,0.499034594258913,-6.02245192508737));
#27221=CARTESIAN_POINT('Ctrl Pts',(53.8378782957208,3.30525812003113,-5.0590741718445));
#27222=CARTESIAN_POINT('Ctrl Pts',(54.3905098746681,5.31474092080006,-2.8761939540005));
#27223=CARTESIAN_POINT('Ctrl Pts',(54.9431414536155,6.0430921485822,-6.36963580352865E-15));
#27224=CARTESIAN_POINT('Ctrl Pts',(55.4957730325629,5.31474092080007,2.8761939540005));
#27225=CARTESIAN_POINT('Ctrl Pts',(56.0484046115103,3.30525812003113,5.05907417184449));
#27226=CARTESIAN_POINT('Ctrl Pts',(56.6010361904576,0.499034594258907,6.02245192508737));
#27227=CARTESIAN_POINT('Ctrl Pts',(57.1536677694049,-2.42748246684176,5.53410260019017));
#27228=CARTESIAN_POINT('Ctrl Pts',(57.7062993483523,-4.7688488164615,3.71174402161431));
#27229=CARTESIAN_POINT('Ctrl Pts',(58.2589309272996,-5.9606722482583,0.994660276224585));
#27230=CARTESIAN_POINT('Ctrl Pts',(58.8115625062471,-5.71566074731474,-1.96218881299959));
#27231=CARTESIAN_POINT('Ctrl Pts',(59.3641940851944,-4.09287494787099,-4.44604738811308));
#27232=CARTESIAN_POINT('Ctrl Pts',(59.9168256641418,-1.4834914199313,-5.85817513593128));
#27233=CARTESIAN_POINT('Ctrl Pts',(60.4694572430892,1.48349141993113,-5.85817513593183));
#27234=CARTESIAN_POINT('Ctrl Pts',(61.0220888220365,4.09287494787156,-4.44604738811222));
#27235=CARTESIAN_POINT('Ctrl Pts',(61.574720400984,5.71566074731343,-1.96218881300128));
#27236=CARTESIAN_POINT('Ctrl Pts',(62.1273519799312,5.96067224826113,0.994660276228038));
#27237=CARTESIAN_POINT('Ctrl Pts',(62.6799835588787,4.76884881645555,3.71174402160707));
#27238=CARTESIAN_POINT('Ctrl Pts',(63.232615137826,2.42748246685427,5.53410260020538));
#27239=CARTESIAN_POINT('Ctrl Pts',(63.7852467167734,-0.499034594285243,
6.02245192505537));
#27240=CARTESIAN_POINT('Ctrl Pts',(64.3378782957207,-3.30525811997573,5.05907417191182));
#27241=CARTESIAN_POINT('Ctrl Pts',(64.8905098746681,-5.31474092091658,2.87619395385889));
#27242=CARTESIAN_POINT('Ctrl Pts',(65.4431414536155,-6.04309214833712,2.97887036704478E-10));
#27243=CARTESIAN_POINT('Ctrl Pts',(65.9957730325628,-5.31474092131558,-2.87619395462708));
#27244=CARTESIAN_POINT('Ctrl Pts',(66.5484046115102,-3.30525811894677,-5.05907417052651));
#27245=CARTESIAN_POINT('Ctrl Pts',(67.1010361904576,-0.499034596539806,
-6.0224519278597));
#27246=CARTESIAN_POINT('Ctrl Pts',(67.653667769405,2.42748247163954,-5.5341025943587));
#27247=CARTESIAN_POINT('Ctrl Pts',(68.2062993483523,4.76884880636957,-3.71174403388056));
#27248=CARTESIAN_POINT('Ctrl Pts',(68.7589309272997,5.96067226948623,-0.994660250423083));
#27249=CARTESIAN_POINT('Ctrl Pts',(69.3115625062471,5.71566070266274,1.96218875872725));
#27250=CARTESIAN_POINT('Ctrl Pts',(69.8641940851944,4.09287504179451,4.44604750227256));
#27251=CARTESIAN_POINT('Ctrl Pts',(70.4168256641419,1.48349122236702,5.85817489580176));
#27252=CARTESIAN_POINT('Ctrl Pts',(70.9694572430892,-1.48349100436534,5.85817564103365));
#27253=CARTESIAN_POINT('Ctrl Pts',(71.5220888220366,-4.09287582201279,4.44604632565119));
#27254=CARTESIAN_POINT('Ctrl Pts',(72.0747204009839,-5.71565890873659,1.96219104782992));
#27255=CARTESIAN_POINT('Ctrl Pts',(72.6273519799313,-5.9606761168237,-0.994664977192599));
#27256=CARTESIAN_POINT('Ctrl Pts',(73.1799835588787,-4.76884068918239,-3.71173413415616));
#27257=CARTESIAN_POINT('Ctrl Pts',(73.732615137826,-2.42749964852484,-5.53412340547436));
#27258=CARTESIAN_POINT('Ctrl Pts',(74.2852467167734,0.499070024096889,-6.02240821551781));
#27259=CARTESIAN_POINT('Ctrl Pts',(74.8378782957208,3.30517718677736,-5.05916675657822));
#27260=CARTESIAN_POINT('Ctrl Pts',(75.3905098746681,5.31486464408031,-2.87600085013837));
#27261=CARTESIAN_POINT('Ctrl Pts',(75.7589309272997,5.79981109503712,-0.958997471436831));
#27262=CARTESIAN_POINT('Ctrl Pts',(75.9431414536155,5.79981109503712,-8.52326411183583E-15));
#27263=CARTESIAN_POINT('Ctrl Pts',(33.62030855087,6.05892730518855,0.));
#27264=CARTESIAN_POINT('Ctrl Pts',(33.8045190771858,6.05892730518855,1.00170122537842));
#27265=CARTESIAN_POINT('Ctrl Pts',(34.1729401298174,5.55226374371841,3.00453419845087));
#27266=CARTESIAN_POINT('Ctrl Pts',(34.7255717087647,3.45282354398353,5.28512205116659));
#27267=CARTESIAN_POINT('Ctrl Pts',(35.2782032877121,0.52135987967838,6.29143885263431));
#27268=CARTESIAN_POINT('Ctrl Pts',(35.8308348666595,-2.53593227701648,5.78132024999939));
#27269=CARTESIAN_POINT('Ctrl Pts',(36.3834664456069,-4.98186108464976,3.87753730806675));
#27270=CARTESIAN_POINT('Ctrl Pts',(36.9360980245542,-6.22693362925883,1.03909408852531));
#27271=CARTESIAN_POINT('Ctrl Pts',(37.4887296035016,-5.97097223597331,-2.04983951271052));
#27272=CARTESIAN_POINT('Ctrl Pts',(38.0413611824489,-4.27570069868504,-4.64464744982032));
#27273=CARTESIAN_POINT('Ctrl Pts',(38.5939927613963,-1.54975720378295,-6.11985471822127));
#27274=CARTESIAN_POINT('Ctrl Pts',(39.1466243403437,1.54975741221459,-6.11985420086809));
#27275=CARTESIAN_POINT('Ctrl Pts',(39.6992559192911,4.27569995271762,-4.64464826665024));
#27276=CARTESIAN_POINT('Ctrl Pts',(40.2518874982384,5.97097395114776,-2.04983792356467));
#27277=CARTESIAN_POINT('Ctrl Pts',(40.8045190771858,6.22692995081589,1.03909080720973));
#27278=CARTESIAN_POINT('Ctrl Pts',(41.3571506561332,4.98186884549998,3.87754418138483));
#27279=CARTESIAN_POINT('Ctrl Pts',(41.9097822350805,2.53591585418045,5.78130580919469));
#27280=CARTESIAN_POINT('Ctrl Pts',(42.4624138140279,-0.521326007358065,
6.29146924994462));
#27281=CARTESIAN_POINT('Ctrl Pts',(43.0150453929753,-3.45290092330605,5.28505830615491));
#27282=CARTESIAN_POINT('Ctrl Pts',(43.5676769719227,-5.55214545226785,3.00467086174248));
#27283=CARTESIAN_POINT('Ctrl Pts',(44.12030855087,-6.31303145085601,-2.06792707167108E-10));
#27284=CARTESIAN_POINT('Ctrl Pts',(44.6729401298174,-5.55214545188636,-3.00467086120918));
#27285=CARTESIAN_POINT('Ctrl Pts',(45.2255717087647,-3.45290092428985,-5.28505830711662));
#27286=CARTESIAN_POINT('Ctrl Pts',(45.7782032877121,-0.521326005202469,
-6.29146924799781));
#27287=CARTESIAN_POINT('Ctrl Pts',(46.3308348666595,2.53591584960525,-5.78130581325357));
#27288=CARTESIAN_POINT('Ctrl Pts',(46.8834664456069,4.98186885514319,-3.87754417286436));
#27289=CARTESIAN_POINT('Ctrl Pts',(47.4360980245542,6.22692993052255,-1.03909082512399));
#27290=CARTESIAN_POINT('Ctrl Pts',(47.9887296035015,5.97097399383832,2.04983796124264));
#27291=CARTESIAN_POINT('Ctrl Pts',(48.541361182449,4.27569986291781,4.64464818739812));
#27292=CARTESIAN_POINT('Ctrl Pts',(49.0939927613963,1.54975760110581,6.11985436757058));
#27293=CARTESIAN_POINT('Ctrl Pts',(49.6466243403437,-1.54975760110596,6.11985436757021));
#27294=CARTESIAN_POINT('Ctrl Pts',(50.199255919291,-4.27569986291726,4.64464818739871));
#27295=CARTESIAN_POINT('Ctrl Pts',(50.7518874982385,-5.97097399383958,2.04983796124148));
#27296=CARTESIAN_POINT('Ctrl Pts',(51.3045190771858,-6.22692993051986,-1.03909082512159));
#27297=CARTESIAN_POINT('Ctrl Pts',(51.8571506561332,-4.98186885514887,-3.87754417286939));
#27298=CARTESIAN_POINT('Ctrl Pts',(52.4097822350806,-2.53591584959328,-5.781305813243));
#27299=CARTESIAN_POINT('Ctrl Pts',(52.9624138140279,0.521326005177292,-6.29146924802002));
#27300=CARTESIAN_POINT('Ctrl Pts',(53.5150453929753,3.45290092434281,-5.28505830706988));
#27301=CARTESIAN_POINT('Ctrl Pts',(54.0676769719227,5.55214545177497,-3.0046708613075));
#27302=CARTESIAN_POINT('Ctrl Pts',(54.62030855087,6.31303145109033,-5.36390383455044E-15));
#27303=CARTESIAN_POINT('Ctrl Pts',(55.1729401298174,5.55214545177497,3.0046708613075));
#27304=CARTESIAN_POINT('Ctrl Pts',(55.7255717087647,3.45290092434281,5.28505830706987));
#27305=CARTESIAN_POINT('Ctrl Pts',(56.2782032877121,0.521326005177289,6.29146924802003));
#27306=CARTESIAN_POINT('Ctrl Pts',(56.8308348666595,-2.5359158495933,5.781305813243));
#27307=CARTESIAN_POINT('Ctrl Pts',(57.3834664456068,-4.98186885514888,3.87754417286939));
#27308=CARTESIAN_POINT('Ctrl Pts',(57.9360980245542,-6.22692993051986,1.03909082512159));
#27309=CARTESIAN_POINT('Ctrl Pts',(58.4887296035016,-5.97097399383958,-2.04983796124148));
#27310=CARTESIAN_POINT('Ctrl Pts',(59.041361182449,-4.27569986291726,-4.64464818739871));
#27311=CARTESIAN_POINT('Ctrl Pts',(59.5939927613963,-1.54975760110596,-6.11985436757021));
#27312=CARTESIAN_POINT('Ctrl Pts',(60.1466243403437,1.5497576011058,-6.11985436757059));
#27313=CARTESIAN_POINT('Ctrl Pts',(60.699255919291,4.2756998629178,-4.64464818739812));
#27314=CARTESIAN_POINT('Ctrl Pts',(61.2518874982385,5.97097399383833,-2.04983796124265));
#27315=CARTESIAN_POINT('Ctrl Pts',(61.8045190771858,6.22692993052255,1.03909082512398));
#27316=CARTESIAN_POINT('Ctrl Pts',(62.3571506561332,4.98186885514319,3.87754417286436));
#27317=CARTESIAN_POINT('Ctrl Pts',(62.9097822350805,2.53591584960525,5.78130581325356));
#27318=CARTESIAN_POINT('Ctrl Pts',(63.4624138140279,-0.521326005202466,
6.2914692479978));
#27319=CARTESIAN_POINT('Ctrl Pts',(64.0150453929752,-3.45290092428985,5.28505830711661));
#27320=CARTESIAN_POINT('Ctrl Pts',(64.5676769719227,-5.55214545188636,3.00467086120919));
#27321=CARTESIAN_POINT('Ctrl Pts',(65.1203085508701,-6.31303145085602,2.06801021218025E-10));
#27322=CARTESIAN_POINT('Ctrl Pts',(65.6729401298174,-5.55214545226785,-3.00467086174248));
#27323=CARTESIAN_POINT('Ctrl Pts',(66.2255717087647,-3.45290092330605,-5.28505830615491));
#27324=CARTESIAN_POINT('Ctrl Pts',(66.7782032877121,-0.521326007358057,
-6.29146924994462));
#27325=CARTESIAN_POINT('Ctrl Pts',(67.3308348666595,2.53591585418046,-5.78130580919469));
#27326=CARTESIAN_POINT('Ctrl Pts',(67.8834664456069,4.98186884549998,-3.87754418138483));
#27327=CARTESIAN_POINT('Ctrl Pts',(68.4360980245542,6.22692995081589,-1.03909080720973));
#27328=CARTESIAN_POINT('Ctrl Pts',(68.9887296035016,5.97097395114776,2.04983792356467));
#27329=CARTESIAN_POINT('Ctrl Pts',(69.541361182449,4.27569995271762,4.64464826665024));
#27330=CARTESIAN_POINT('Ctrl Pts',(70.0939927613963,1.54975741221458,6.1198542008681));
#27331=CARTESIAN_POINT('Ctrl Pts',(70.6466243403438,-1.54975720378297,6.11985471822127));
#27332=CARTESIAN_POINT('Ctrl Pts',(71.199255919291,-4.27570069868505,4.6446474498203));
#27333=CARTESIAN_POINT('Ctrl Pts',(71.7518874982385,-5.9709722359733,2.04983951271053));
#27334=CARTESIAN_POINT('Ctrl Pts',(72.3045190771858,-6.22693362925883,-1.03909408852532));
#27335=CARTESIAN_POINT('Ctrl Pts',(72.8571506561333,-4.98186108464976,-3.87753730806676));
#27336=CARTESIAN_POINT('Ctrl Pts',(73.4097822350805,-2.53593227701648,-5.78132024999937));
#27337=CARTESIAN_POINT('Ctrl Pts',(73.962413814028,0.521359879678368,-6.29143885263431));
#27338=CARTESIAN_POINT('Ctrl Pts',(74.5150453929753,3.45282354398353,-5.2851220511666));
#27339=CARTESIAN_POINT('Ctrl Pts',(75.0676769719227,5.55226374371841,-3.00453419845087));
#27340=CARTESIAN_POINT('Ctrl Pts',(75.4360980245542,6.05892730518855,-1.00170122537842));
#27341=CARTESIAN_POINT('Ctrl Pts',(75.62030855087,6.05892730518855,-8.90405511667878E-15));
#27342=CARTESIAN_POINT('Ctrl Pts',(33.1358237202237,5.94680344913766,0.));
#27343=CARTESIAN_POINT('Ctrl Pts',(33.3200342465395,5.94680344913766,0.983379197578396));
#27344=CARTESIAN_POINT('Ctrl Pts',(33.6884552991711,5.44959421336945,2.94886771297254));
#27345=CARTESIAN_POINT('Ctrl Pts',(34.2410868781184,3.38895443893944,5.18742673184628));
#27346=CARTESIAN_POINT('Ctrl Pts',(34.7937184570658,0.511722382884761,6.17505868653612));
#27347=CARTESIAN_POINT('Ctrl Pts',(35.3463500360132,-2.48903384632581,5.67440885923965));
#27348=CARTESIAN_POINT('Ctrl Pts',(35.8989816149605,-4.88972305399822,3.80581898848347));
#27349=CARTESIAN_POINT('Ctrl Pts',(36.4516131939079,-6.11177024810298,1.01987909450271));
#27350=CARTESIAN_POINT('Ctrl Pts',(37.0042447728553,-5.86054195732468,-2.01192998939814));
#27351=CARTESIAN_POINT('Ctrl Pts',(37.5568763518026,-4.19662395290879,-4.55874653989111));
#27352=CARTESIAN_POINT('Ctrl Pts',(38.10950793075,-1.52109519307483,-6.00667145344936));
#27353=CARTESIAN_POINT('Ctrl Pts',(38.6621395096974,1.5210954270842,-6.00667054754812));
#27354=CARTESIAN_POINT('Ctrl Pts',(39.2147710886447,4.19662311539983,-4.55874797018865));
#27355=CARTESIAN_POINT('Ctrl Pts',(39.7674026675921,5.86054388297712,-2.01192720677863));
#27356=CARTESIAN_POINT('Ctrl Pts',(40.3200342465395,6.11176611825916,1.01987334860882));
#27357=CARTESIAN_POINT('Ctrl Pts',(40.8726658254868,4.88973176722276,3.80583102214387));
#27358=CARTESIAN_POINT('Ctrl Pts',(41.4252974044342,2.4890154081581,5.67438355771667));
#27359=CARTESIAN_POINT('Ctrl Pts',(41.9779289833816,-0.511684353915735,
6.17511179518466));
#27360=CARTESIAN_POINT('Ctrl Pts',(42.5305605623289,-3.38904131388133,5.18731389692575));
#27361=CARTESIAN_POINT('Ctrl Pts',(43.0831921412763,-5.44946140575937,2.9491010349948));
#27362=CARTESIAN_POINT('Ctrl Pts',(43.6358237202237,-6.19627521287463,-3.62104274501345E-10));
#27363=CARTESIAN_POINT('Ctrl Pts',(44.1884552991711,-5.44946140533107,-2.94910103406097));
#27364=CARTESIAN_POINT('Ctrl Pts',(44.7410868781184,-3.38904131498586,-5.18731389860973));
#27365=CARTESIAN_POINT('Ctrl Pts',(45.2937184570658,-0.511684351495615,
-6.17511179177572));
#27366=CARTESIAN_POINT('Ctrl Pts',(45.8463500360132,2.48901540302145,-5.67438356482389));
#27367=CARTESIAN_POINT('Ctrl Pts',(46.3989816149605,4.88973177804935,-3.80583100722426));
#27368=CARTESIAN_POINT('Ctrl Pts',(46.9516131939079,6.11176609547551,-1.01987337997725));
#27369=CARTESIAN_POINT('Ctrl Pts',(47.5042447728553,5.86054393090647,2.01192727275394));
#27370=CARTESIAN_POINT('Ctrl Pts',(48.0568763518026,4.19662301458021,4.55874783141572));
#27371=CARTESIAN_POINT('Ctrl Pts',(48.60950793075,1.52109563915525,6.00667083944942));
#27372=CARTESIAN_POINT('Ctrl Pts',(49.1621395096974,-1.52109563915541,6.00667083944875));
#27373=CARTESIAN_POINT('Ctrl Pts',(49.7147710886447,-4.1966230145796,4.55874783141676));
#27374=CARTESIAN_POINT('Ctrl Pts',(50.2674026675921,-5.86054393090788,2.0119272727519));
#27375=CARTESIAN_POINT('Ctrl Pts',(50.8200342465394,-6.1117660954725,-1.01987337997305));
#27376=CARTESIAN_POINT('Ctrl Pts',(51.3726658254868,-4.88973177805572,-3.80583100723307));
#27377=CARTESIAN_POINT('Ctrl Pts',(51.9252974044342,-2.48901540300802,-5.67438356480538));
#27378=CARTESIAN_POINT('Ctrl Pts',(52.4779289833816,0.511684351467352,-6.17511179181463));
#27379=CARTESIAN_POINT('Ctrl Pts',(53.030560562329,3.38904131504531,-5.18731389852789));
#27380=CARTESIAN_POINT('Ctrl Pts',(53.5831921412763,5.449461405206,-2.94910103423313));
#27381=CARTESIAN_POINT('Ctrl Pts',(54.1358237202237,6.1962752131377,-6.168489409733E-15));
#27382=CARTESIAN_POINT('Ctrl Pts',(54.688455299171,5.44946140520601,2.94910103423312));
#27383=CARTESIAN_POINT('Ctrl Pts',(55.2410868781184,3.38904131504531,5.18731389852788));
#27384=CARTESIAN_POINT('Ctrl Pts',(55.7937184570658,0.511684351467345,6.17511179181463));
#27385=CARTESIAN_POINT('Ctrl Pts',(56.3463500360131,-2.48901540300803,5.67438356480538));
#27386=CARTESIAN_POINT('Ctrl Pts',(56.8989816149606,-4.88973177805573,3.80583100723306));
#27387=CARTESIAN_POINT('Ctrl Pts',(57.4516131939078,-6.1117660954725,1.01987337997304));
#27388=CARTESIAN_POINT('Ctrl Pts',(58.0042447728553,-5.86054393090788,-2.0119272727519));
#27389=CARTESIAN_POINT('Ctrl Pts',(58.5568763518026,-4.1966230145796,-4.55874783141676));
#27390=CARTESIAN_POINT('Ctrl Pts',(59.1095079307501,-1.52109563915542,-6.00667083944875));
#27391=CARTESIAN_POINT('Ctrl Pts',(59.6621395096973,1.52109563915524,-6.00667083944942));
#27392=CARTESIAN_POINT('Ctrl Pts',(60.2147710886447,4.1966230145802,-4.55874783141572));
#27393=CARTESIAN_POINT('Ctrl Pts',(60.7674026675922,5.86054393090647,-2.01192727275395));
#27394=CARTESIAN_POINT('Ctrl Pts',(61.3200342465394,6.11176609547552,1.01987337997724));
#27395=CARTESIAN_POINT('Ctrl Pts',(61.8726658254869,4.88973177804935,3.80583100722426));
#27396=CARTESIAN_POINT('Ctrl Pts',(62.4252974044342,2.48901540302145,5.67438356482389));
#27397=CARTESIAN_POINT('Ctrl Pts',(62.9779289833816,-0.511684351495617,
6.17511179177572));
#27398=CARTESIAN_POINT('Ctrl Pts',(63.5305605623289,-3.38904131498585,5.18731389860973));
#27399=CARTESIAN_POINT('Ctrl Pts',(64.0831921412763,-5.44946140533107,2.94910103406098));
#27400=CARTESIAN_POINT('Ctrl Pts',(64.6358237202237,-6.19627521287463,3.62109504307536E-10));
#27401=CARTESIAN_POINT('Ctrl Pts',(65.188455299171,-5.44946140575937,-2.94910103499479));
#27402=CARTESIAN_POINT('Ctrl Pts',(65.7410868781184,-3.38904131388132,-5.18731389692575));
#27403=CARTESIAN_POINT('Ctrl Pts',(66.2937184570658,-0.511684353915733,
-6.17511179518466));
#27404=CARTESIAN_POINT('Ctrl Pts',(66.8463500360131,2.48901540815811,-5.67438355771667));
#27405=CARTESIAN_POINT('Ctrl Pts',(67.3989816149605,4.88973176722276,-3.80583102214386));
#27406=CARTESIAN_POINT('Ctrl Pts',(67.9516131939078,6.11176611825917,-1.01987334860882));
#27407=CARTESIAN_POINT('Ctrl Pts',(68.5042447728553,5.86054388297712,2.01192720677863));
#27408=CARTESIAN_POINT('Ctrl Pts',(69.0568763518026,4.19662311539983,4.55874797018865));
#27409=CARTESIAN_POINT('Ctrl Pts',(69.60950793075,1.52109542708419,6.00667054754813));
#27410=CARTESIAN_POINT('Ctrl Pts',(70.1621395096974,-1.52109519307484,6.00667145344936));
#27411=CARTESIAN_POINT('Ctrl Pts',(70.7147710886448,-4.19662395290879,4.5587465398911));
#27412=CARTESIAN_POINT('Ctrl Pts',(71.2674026675922,-5.86054195732468,2.01192998939814));
#27413=CARTESIAN_POINT('Ctrl Pts',(71.8200342465394,-6.11177024810298,-1.01987909450272));
#27414=CARTESIAN_POINT('Ctrl Pts',(72.3726658254869,-4.88972305399822,-3.80581898848348));
#27415=CARTESIAN_POINT('Ctrl Pts',(72.9252974044342,-2.48903384632581,-5.67440885923964));
#27416=CARTESIAN_POINT('Ctrl Pts',(73.4779289833816,0.511722382884753,-6.17505868653612));
#27417=CARTESIAN_POINT('Ctrl Pts',(74.0305605623289,3.38895443893944,-5.18742673184629));
#27418=CARTESIAN_POINT('Ctrl Pts',(74.5831921412763,5.44959421336945,-2.94886771297254));
#27419=CARTESIAN_POINT('Ctrl Pts',(74.9516131939079,5.94680344913766,-0.983379197578397));
#27420=CARTESIAN_POINT('Ctrl Pts',(75.1358237202237,5.94680344913766,-8.73928057097385E-15));
#27421=CARTESIAN_POINT('Ctrl Pts',(32.9926516271063,5.64959965017094,0.));
#27422=CARTESIAN_POINT('Ctrl Pts',(33.1768621534221,5.64959965017094,0.934105498328347));
#27423=CARTESIAN_POINT('Ctrl Pts',(33.5452832060536,5.17719316068765,2.80153095913731));
#27424=CARTESIAN_POINT('Ctrl Pts',(34.097914785001,3.21956825042242,4.92810992359527));
#27425=CARTESIAN_POINT('Ctrl Pts',(34.6505463639483,0.486141746602274,5.86641986341936));
#27426=CARTESIAN_POINT('Ctrl Pts',(35.2031779428958,-2.36462122333319,5.39077403004133));
#27427=CARTESIAN_POINT('Ctrl Pts',(35.7558095218431,-4.64531700059631,3.61559300345088));
#27428=CARTESIAN_POINT('Ctrl Pts',(36.3084411007905,-5.80628073241482,0.968900224297807));
#27429=CARTESIAN_POINT('Ctrl Pts',(36.8610726797378,-5.56761023028957,-1.91136547361583));
#27430=CARTESIAN_POINT('Ctrl Pts',(37.4137042586852,-3.98686087342849,-4.33088362081724));
#27431=CARTESIAN_POINT('Ctrl Pts',(37.9663358376326,-1.44506518185627,-5.7064353192738));
#27432=CARTESIAN_POINT('Ctrl Pts',(38.5189674165799,1.445065386745,-5.7064346943363));
#27433=CARTESIAN_POINT('Ctrl Pts',(39.0715989955273,3.98686014014099,-4.33088460750931));
#27434=CARTESIAN_POINT('Ctrl Pts',(39.6242305744747,5.56761191630958,-1.91136355401326));
#27435=CARTESIAN_POINT('Ctrl Pts',(40.1768621534221,5.80627711649786,0.968896260552868));
#27436=CARTESIAN_POINT('Ctrl Pts',(40.7294937323694,4.64532462952802,3.61560130546583));
#27437=CARTESIAN_POINT('Ctrl Pts',(41.2821253113168,2.36460507965162,5.39075658079754));
#27438=CARTESIAN_POINT('Ctrl Pts',(41.8347568902642,-0.486108450041791,
5.86645653965694));
#27439=CARTESIAN_POINT('Ctrl Pts',(42.3873884692115,-3.21964431445548,4.92803248756168));
#27440=CARTESIAN_POINT('Ctrl Pts',(42.9400200481589,-5.17707687994863,2.80169390094401));
#27441=CARTESIAN_POINT('Ctrl Pts',(43.4926516271062,-5.88656213122846,-2.49796196989472E-10));
#27442=CARTESIAN_POINT('Ctrl Pts',(44.0452832060537,-5.17707687957364,-2.80169390029981));
#27443=CARTESIAN_POINT('Ctrl Pts',(44.597914785001,-3.21964431542256,-4.92803248872338));
#27444=CARTESIAN_POINT('Ctrl Pts',(45.1505463639484,-0.486108447922835,
-5.86645653730528));
#27445=CARTESIAN_POINT('Ctrl Pts',(45.7031779428957,2.36460507515419,-5.39075658570046));
#27446=CARTESIAN_POINT('Ctrl Pts',(46.2558095218431,4.64532463900732,-3.61560129517351));
#27447=CARTESIAN_POINT('Ctrl Pts',(46.8084411007904,5.80627709654946,-0.968896282192427));
#27448=CARTESIAN_POINT('Ctrl Pts',(47.3610726797379,5.5676119582745,1.91136359952644));
#27449=CARTESIAN_POINT('Ctrl Pts',(47.9137042586852,3.98686005186758,4.33088451177657));
#27450=CARTESIAN_POINT('Ctrl Pts',(48.4663358376326,1.44506557242546,5.70643489570486));
#27451=CARTESIAN_POINT('Ctrl Pts',(49.0189674165799,-1.4450655724256,5.7064348957044));
#27452=CARTESIAN_POINT('Ctrl Pts',(49.5715989955273,-3.98686005186705,4.3308845117773));
#27453=CARTESIAN_POINT('Ctrl Pts',(50.1242305744747,-5.56761195827573,1.91136359952503));
#27454=CARTESIAN_POINT('Ctrl Pts',(50.6768621534221,-5.80627709654682,-0.968896282189531));
#27455=CARTESIAN_POINT('Ctrl Pts',(51.2294937323694,-4.6453246390129,-3.61560129517959));
#27456=CARTESIAN_POINT('Ctrl Pts',(51.7821253113168,-2.36460507514243,-5.3907565856877));
#27457=CARTESIAN_POINT('Ctrl Pts',(52.3347568902641,0.486108447898087,-5.86645653733213));
#27458=CARTESIAN_POINT('Ctrl Pts',(52.8873884692115,3.21964431547462,-4.92803248866692));
#27459=CARTESIAN_POINT('Ctrl Pts',(53.4400200481589,5.17707687946413,-2.80169390041857));
#27460=CARTESIAN_POINT('Ctrl Pts',(53.9926516271062,5.88656213145879,-3.62063508832155E-15));
#27461=CARTESIAN_POINT('Ctrl Pts',(54.5452832060537,5.17707687946413,2.80169390041857));
#27462=CARTESIAN_POINT('Ctrl Pts',(55.0979147850009,3.21964431547461,4.92803248866692));
#27463=CARTESIAN_POINT('Ctrl Pts',(55.6505463639484,0.486108447898084,5.86645653733212));
#27464=CARTESIAN_POINT('Ctrl Pts',(56.2031779428957,-2.36460507514244,5.3907565856877));
#27465=CARTESIAN_POINT('Ctrl Pts',(56.7558095218431,-4.64532463901291,3.61560129517958));
#27466=CARTESIAN_POINT('Ctrl Pts',(57.3084411007904,-5.80627709654682,0.968896282189525));
#27467=CARTESIAN_POINT('Ctrl Pts',(57.8610726797378,-5.56761195827573,-1.91136359952503));
#27468=CARTESIAN_POINT('Ctrl Pts',(58.4137042586852,-3.98686005186705,-4.3308845117773));
#27469=CARTESIAN_POINT('Ctrl Pts',(58.9663358376325,-1.44506557242561,-5.7064348957044));
#27470=CARTESIAN_POINT('Ctrl Pts',(59.51896741658,1.44506557242545,-5.70643489570486));
#27471=CARTESIAN_POINT('Ctrl Pts',(60.0715989955273,3.98686005186758,-4.33088451177658));
#27472=CARTESIAN_POINT('Ctrl Pts',(60.6242305744747,5.5676119582745,-1.91136359952644));
#27473=CARTESIAN_POINT('Ctrl Pts',(61.176862153422,5.80627709654946,0.968896282192422));
#27474=CARTESIAN_POINT('Ctrl Pts',(61.7294937323694,4.64532463900732,3.61560129517351));
#27475=CARTESIAN_POINT('Ctrl Pts',(62.2821253113167,2.36460507515419,5.39075658570046));
#27476=CARTESIAN_POINT('Ctrl Pts',(62.8347568902642,-0.486108447922834,
5.86645653730528));
#27477=CARTESIAN_POINT('Ctrl Pts',(63.3873884692115,-3.21964431542255,4.92803248872338));
#27478=CARTESIAN_POINT('Ctrl Pts',(63.9400200481589,-5.17707687957363,2.80169390029982));
#27479=CARTESIAN_POINT('Ctrl Pts',(64.4926516271063,-5.88656213122846,2.49803438259616E-10));
#27480=CARTESIAN_POINT('Ctrl Pts',(65.0452832060536,-5.17707687994864,-2.80169390094401));
#27481=CARTESIAN_POINT('Ctrl Pts',(65.597914785001,-3.21964431445548,-4.92803248756169));
#27482=CARTESIAN_POINT('Ctrl Pts',(66.1505463639484,-0.486108450041783,
-5.86645653965694));
#27483=CARTESIAN_POINT('Ctrl Pts',(66.7031779428957,2.36460507965163,-5.39075658079754));
#27484=CARTESIAN_POINT('Ctrl Pts',(67.255809521843,4.64532462952802,-3.61560130546582));
#27485=CARTESIAN_POINT('Ctrl Pts',(67.8084411007905,5.80627711649786,-0.96889626055287));
#27486=CARTESIAN_POINT('Ctrl Pts',(68.3610726797379,5.56761191630958,1.91136355401326));
#27487=CARTESIAN_POINT('Ctrl Pts',(68.9137042586851,3.98686014014099,4.33088460750931));
#27488=CARTESIAN_POINT('Ctrl Pts',(69.4663358376326,1.44506538674499,5.7064346943363));
#27489=CARTESIAN_POINT('Ctrl Pts',(70.0189674165799,-1.44506518185629,5.7064353192738));
#27490=CARTESIAN_POINT('Ctrl Pts',(70.5715989955273,-3.98686087342849,4.33088362081724));
#27491=CARTESIAN_POINT('Ctrl Pts',(71.1242305744747,-5.56761023028957,1.91136547361582));
#27492=CARTESIAN_POINT('Ctrl Pts',(71.6768621534221,-5.80628073241483,-0.968900224297809));
#27493=CARTESIAN_POINT('Ctrl Pts',(72.2294937323694,-4.64531700059631,-3.61559300345089));
#27494=CARTESIAN_POINT('Ctrl Pts',(72.7821253113168,-2.36462122333319,-5.39077403004132));
#27495=CARTESIAN_POINT('Ctrl Pts',(73.3347568902641,0.486141746602262,-5.86641986341937));
#27496=CARTESIAN_POINT('Ctrl Pts',(73.8873884692115,3.21956825042242,-4.92810992359527));
#27497=CARTESIAN_POINT('Ctrl Pts',(74.4400200481589,5.17719316068764,-2.80153095913731));
#27498=CARTESIAN_POINT('Ctrl Pts',(74.8084411007905,5.64959965017094,-0.934105498328348));
#27499=CARTESIAN_POINT('Ctrl Pts',(74.9926516271063,5.64959965017094,-8.30251695365502E-15));
#27500=CARTESIAN_POINT('Ctrl Pts',(32.9926516271063,5.35040034982906,0.));
#27501=CARTESIAN_POINT('Ctrl Pts',(33.1768621534221,5.35040034982906,0.884711999783592));
#27502=CARTESIAN_POINT('Ctrl Pts',(33.5452832060536,4.90303992219514,2.65314027768598));
#27503=CARTESIAN_POINT('Ctrl Pts',(34.097914785001,3.04907159007201,4.66715881783104));
#27504=CARTESIAN_POINT('Ctrl Pts',(34.6505463639483,0.460399720877627,5.55575434845313));
#27505=CARTESIAN_POINT('Ctrl Pts',(35.2031779428958,-2.23940312125801,5.10530860391639));
#27506=CARTESIAN_POINT('Ctrl Pts',(35.7558095218431,-4.39932305117563,3.42412678374845));
#27507=CARTESIAN_POINT('Ctrl Pts',(36.3084411007905,-5.49880832246205,0.917592835722961));
#27508=CARTESIAN_POINT('Ctrl Pts',(36.8610726797378,-5.272776384942,-1.81014920900501));
#27509=CARTESIAN_POINT('Ctrl Pts',(37.4137042586852,-3.77573601188937,-4.10154073270038));
#27510=CARTESIAN_POINT('Ctrl Pts',(37.9663358376326,-1.36854148671349,-5.40425015093622));
#27511=CARTESIAN_POINT('Ctrl Pts',(38.5189674165799,1.36854169117612,-5.40424941809581));
#27512=CARTESIAN_POINT('Ctrl Pts',(39.0715989955273,3.77573528012686,-4.1015418897575));
#27513=CARTESIAN_POINT('Ctrl Pts',(39.6242305744747,5.27277806745566,-1.81014695796662));
#27514=CARTESIAN_POINT('Ctrl Pts',(40.1768621534221,5.49880471406498,0.917588187532836));
#27515=CARTESIAN_POINT('Ctrl Pts',(40.7294937323694,4.39933066424171,3.42413651873231));
#27516=CARTESIAN_POINT('Ctrl Pts',(41.2821253113168,2.23938701114991,5.10528813768847));
#27517=CARTESIAN_POINT('Ctrl Pts',(41.8347568902642,-0.460366493562869,
5.55579732502866));
#27518=CARTESIAN_POINT('Ctrl Pts',(42.3873884692115,-3.04914749591728,4.66706767925751));
#27519=CARTESIAN_POINT('Ctrl Pts',(42.9400200481589,-4.90292388328124,2.65332971861579));
#27520=CARTESIAN_POINT('Ctrl Pts',(43.4926516271062,-5.57483822100387,-2.9292627494233E-10));
#27521=CARTESIAN_POINT('Ctrl Pts',(44.0452832060537,-4.90292388290702,-2.65332971786037));
#27522=CARTESIAN_POINT('Ctrl Pts',(44.597914785001,-3.04914749688235,-4.66706768061979));
#27523=CARTESIAN_POINT('Ctrl Pts',(45.1505463639484,-0.460366491448323,
-5.55579732227095));
#27524=CARTESIAN_POINT('Ctrl Pts',(45.7031779428957,2.23938700666183,-5.10528814343794));
#27525=CARTESIAN_POINT('Ctrl Pts',(46.2558095218431,4.3993306737013,-3.4241365066629));
#27526=CARTESIAN_POINT('Ctrl Pts',(46.8084411007904,5.49880469415807,-0.917588212908723));
#27527=CARTESIAN_POINT('Ctrl Pts',(47.3610726797379,5.2727781093333,1.81014701133818));
#27528=CARTESIAN_POINT('Ctrl Pts',(47.9137042586852,3.77573519203703,4.10154177749537));
#27529=CARTESIAN_POINT('Ctrl Pts',(48.4663358376326,1.36854187647043,5.40424965423309));
#27530=CARTESIAN_POINT('Ctrl Pts',(49.0189674165799,-1.36854187647057,5.40424965423255));
#27531=CARTESIAN_POINT('Ctrl Pts',(49.5715989955273,-3.7757351920365,4.10154177749621));
#27532=CARTESIAN_POINT('Ctrl Pts',(50.1242305744747,-5.27277810933453,1.81014701133654));
#27533=CARTESIAN_POINT('Ctrl Pts',(50.6768621534221,-5.49880469415544,-0.917588212905327));
#27534=CARTESIAN_POINT('Ctrl Pts',(51.2294937323694,-4.39933067370686,-3.42413650667002));
#27535=CARTESIAN_POINT('Ctrl Pts',(51.7821253113168,-2.23938700665009,-5.10528814342298));
#27536=CARTESIAN_POINT('Ctrl Pts',(52.3347568902641,0.460366491423626,-5.55579732230242));
#27537=CARTESIAN_POINT('Ctrl Pts',(52.8873884692115,3.0491474969343,-4.66706768055358));
#27538=CARTESIAN_POINT('Ctrl Pts',(53.4400200481589,4.90292388279774,-2.65332971799963));
#27539=CARTESIAN_POINT('Ctrl Pts',(53.9926516271062,5.57483822123373,-6.57078219732429E-15));
#27540=CARTESIAN_POINT('Ctrl Pts',(54.5452832060537,4.90292388279775,2.65332971799963));
#27541=CARTESIAN_POINT('Ctrl Pts',(55.0979147850009,3.0491474969343,4.66706768055358));
#27542=CARTESIAN_POINT('Ctrl Pts',(55.6505463639484,0.460366491423622,5.55579732230243));
#27543=CARTESIAN_POINT('Ctrl Pts',(56.2031779428957,-2.2393870066501,5.10528814342297));
#27544=CARTESIAN_POINT('Ctrl Pts',(56.7558095218432,-4.39933067370687,3.42413650667002));
#27545=CARTESIAN_POINT('Ctrl Pts',(57.3084411007904,-5.49880469415543,0.917588212905322));
#27546=CARTESIAN_POINT('Ctrl Pts',(57.8610726797378,-5.27277810933453,-1.81014701133654));
#27547=CARTESIAN_POINT('Ctrl Pts',(58.4137042586852,-3.7757351920365,-4.10154177749621));
#27548=CARTESIAN_POINT('Ctrl Pts',(58.9663358376325,-1.36854187647058,-5.40424965423255));
#27549=CARTESIAN_POINT('Ctrl Pts',(59.51896741658,1.36854187647042,-5.40424965423309));
#27550=CARTESIAN_POINT('Ctrl Pts',(60.0715989955273,3.77573519203703,-4.10154177749537));
#27551=CARTESIAN_POINT('Ctrl Pts',(60.6242305744747,5.2727781093333,-1.81014701133819));
#27552=CARTESIAN_POINT('Ctrl Pts',(61.176862153422,5.49880469415808,0.917588212908717));
#27553=CARTESIAN_POINT('Ctrl Pts',(61.7294937323694,4.39933067370129,3.4241365066629));
#27554=CARTESIAN_POINT('Ctrl Pts',(62.2821253113167,2.23938700666183,5.10528814343794));
#27555=CARTESIAN_POINT('Ctrl Pts',(62.8347568902642,-0.460366491448322,
5.55579732227095));
#27556=CARTESIAN_POINT('Ctrl Pts',(63.3873884692115,-3.04914749688234,4.66706768061979));
#27557=CARTESIAN_POINT('Ctrl Pts',(63.9400200481589,-4.90292388290702,2.65332971786038));
#27558=CARTESIAN_POINT('Ctrl Pts',(64.4926516271063,-5.57483822100388,2.92934052602853E-10));
#27559=CARTESIAN_POINT('Ctrl Pts',(65.0452832060536,-4.90292388328124,-2.65332971861579));
#27560=CARTESIAN_POINT('Ctrl Pts',(65.597914785001,-3.04914749591728,-4.66706767925751));
#27561=CARTESIAN_POINT('Ctrl Pts',(66.1505463639483,-0.460366493562863,
-5.55579732502866));
#27562=CARTESIAN_POINT('Ctrl Pts',(66.7031779428957,2.23938701114991,-5.10528813768846));
#27563=CARTESIAN_POINT('Ctrl Pts',(67.2558095218431,4.39933066424171,-3.4241365187323));
#27564=CARTESIAN_POINT('Ctrl Pts',(67.8084411007905,5.49880471406499,-0.917588187532837));
#27565=CARTESIAN_POINT('Ctrl Pts',(68.3610726797379,5.27277806745566,1.81014695796662));
#27566=CARTESIAN_POINT('Ctrl Pts',(68.9137042586851,3.77573528012686,4.1015418897575));
#27567=CARTESIAN_POINT('Ctrl Pts',(69.4663358376326,1.36854169117611,5.40424941809582));
#27568=CARTESIAN_POINT('Ctrl Pts',(70.0189674165799,-1.36854148671351,5.40425015093621));
#27569=CARTESIAN_POINT('Ctrl Pts',(70.5715989955273,-3.77573601188937,4.10154073270038));
#27570=CARTESIAN_POINT('Ctrl Pts',(71.1242305744747,-5.272776384942,1.81014920900501));
#27571=CARTESIAN_POINT('Ctrl Pts',(71.6768621534221,-5.49880832246205,-0.917592835722964));
#27572=CARTESIAN_POINT('Ctrl Pts',(72.2294937323694,-4.39932305117562,-3.42412678374846));
#27573=CARTESIAN_POINT('Ctrl Pts',(72.7821253113168,-2.23940312125801,-5.10530860391638));
#27574=CARTESIAN_POINT('Ctrl Pts',(73.3347568902641,0.460399720877618,-5.55575434845314));
#27575=CARTESIAN_POINT('Ctrl Pts',(73.8873884692115,3.04907159007201,-4.66715881783104));
#27576=CARTESIAN_POINT('Ctrl Pts',(74.4400200481589,4.90303992219514,-2.65314027768598));
#27577=CARTESIAN_POINT('Ctrl Pts',(74.8084411007905,5.35040034982906,-0.884711999783593));
#27578=CARTESIAN_POINT('Ctrl Pts',(74.9926516271063,5.35040034982906,-7.86282079509004E-15));
#27579=CARTESIAN_POINT('Ctrl Pts',(33.1358791011789,5.05215470582044,0.));
#27580=CARTESIAN_POINT('Ctrl Pts',(33.3200896274947,5.05215470582044,0.835439667818526));
#27581=CARTESIAN_POINT('Ctrl Pts',(33.6885106801263,4.62974731329617,2.50523368528442));
#27582=CARTESIAN_POINT('Ctrl Pts',(34.2411422590737,2.87911375329489,4.40702109952745));
#27583=CARTESIAN_POINT('Ctrl Pts',(34.793773838021,0.43473796291613,5.24607120227223));
#27584=CARTESIAN_POINT('Ctrl Pts',(35.3464054169684,-2.11457900308638,4.8207403763615));
#27585=CARTESIAN_POINT('Ctrl Pts',(35.8990369959157,-4.15410404637352,3.23326447896726));
#27586=CARTESIAN_POINT('Ctrl Pts',(36.4516685748631,-5.19230421072891,0.866446616436196));
#27587=CARTESIAN_POINT('Ctrl Pts',(37.0043001538105,-4.9788711625536,-1.70925152427458));
#27588=CARTESIAN_POINT('Ctrl Pts',(37.5569317327579,-3.56527606954637,-3.87292025722597));
#27589=CARTESIAN_POINT('Ctrl Pts',(38.1095633117052,-1.29225881290354,-5.10301667120488));
#27590=CARTESIAN_POINT('Ctrl Pts',(38.6621948906526,1.29225901197644,-5.10301589795954));
#27591=CARTESIAN_POINT('Ctrl Pts',(39.2148264696,3.56527535707347,-3.87292147807751));
#27592=CARTESIAN_POINT('Ctrl Pts',(39.7674580485474,4.97887280071541,-1.70924914912885));
#27593=CARTESIAN_POINT('Ctrl Pts',(40.3200896274947,5.19230069745088,0.8664417119428));
#27594=CARTESIAN_POINT('Ctrl Pts',(40.8727212064421,4.15411145875562,3.23327475046642));
#27595=CARTESIAN_POINT('Ctrl Pts',(41.4253527853894,2.11456331764827,4.82071877979622));
#27596=CARTESIAN_POINT('Ctrl Pts',(41.9779843643368,-0.434705611488933,
5.24611653333821));
#27597=CARTESIAN_POINT('Ctrl Pts',(42.5306159432842,-2.87918765822658,4.40692478140854));
#27598=CARTESIAN_POINT('Ctrl Pts',(43.0832475222315,-4.62963433322232,2.50543281017431));
#27599=CARTESIAN_POINT('Ctrl Pts',(43.6358791011789,-5.26409608723815,-3.09079671340081E-10));
#27600=CARTESIAN_POINT('Ctrl Pts',(44.1885106801263,-4.62963433285796,-2.50543280937723));
#27601=CARTESIAN_POINT('Ctrl Pts',(44.7411422590737,-2.87918765916621,-4.40692478284593));
#27602=CARTESIAN_POINT('Ctrl Pts',(45.293773838021,-0.434705609430123,-5.24611653042846));
#27603=CARTESIAN_POINT('Ctrl Pts',(45.8464054169684,2.1145633132785,-4.82071878586269));
#27604=CARTESIAN_POINT('Ctrl Pts',(46.3990369959157,4.15411146796585,-3.23327473773157));
#27605=CARTESIAN_POINT('Ctrl Pts',(46.9516685748631,5.19230067806873,-0.866441738717781));
#27606=CARTESIAN_POINT('Ctrl Pts',(47.5043001538105,4.97887284148914,1.70924920544305));
#27607=CARTESIAN_POINT('Ctrl Pts',(48.0569317327578,3.56527527130573,3.87292135962583));
#27608=CARTESIAN_POINT('Ctrl Pts',(48.6095633117053,1.2922591923863,5.10301614711619));
#27609=CARTESIAN_POINT('Ctrl Pts',(49.1621948906526,-1.29225919238644,5.10301614711562));
#27610=CARTESIAN_POINT('Ctrl Pts',(49.7148264696,-3.56527527130521,3.87292135962672));
#27611=CARTESIAN_POINT('Ctrl Pts',(50.2674580485474,-4.97887284149034,1.70924920544131));
#27612=CARTESIAN_POINT('Ctrl Pts',(50.8200896274947,-5.19230067806616,-0.866441738714198));
#27613=CARTESIAN_POINT('Ctrl Pts',(51.3727212064421,-4.15411146797128,-3.23327473773908));
#27614=CARTESIAN_POINT('Ctrl Pts',(51.9253527853894,-2.11456331326706,-4.8207187858469));
#27615=CARTESIAN_POINT('Ctrl Pts',(52.4779843643368,0.434705609406076,-5.24611653046166));
#27616=CARTESIAN_POINT('Ctrl Pts',(53.0306159432842,2.87918765921679,-4.40692478277608));
#27617=CARTESIAN_POINT('Ctrl Pts',(53.5832475222316,4.62963433275156,-2.50543280952418));
#27618=CARTESIAN_POINT('Ctrl Pts',(54.1358791011789,5.26409608746195,-1.74326874622889E-15));
#27619=CARTESIAN_POINT('Ctrl Pts',(54.6885106801263,4.62963433275157,2.50543280952417));
#27620=CARTESIAN_POINT('Ctrl Pts',(55.2411422590736,2.87918765921679,4.40692478277608));
#27621=CARTESIAN_POINT('Ctrl Pts',(55.793773838021,0.434705609406073,5.24611653046167));
#27622=CARTESIAN_POINT('Ctrl Pts',(56.3464054169684,-2.11456331326707,4.82071878584689));
#27623=CARTESIAN_POINT('Ctrl Pts',(56.8990369959158,-4.15411146797128,3.23327473773908));
#27624=CARTESIAN_POINT('Ctrl Pts',(57.4516685748631,-5.19230067806616,0.866441738714194));
#27625=CARTESIAN_POINT('Ctrl Pts',(58.0043001538105,-4.97887284149034,-1.70924920544131));
#27626=CARTESIAN_POINT('Ctrl Pts',(58.5569317327579,-3.56527527130521,-3.87292135962672));
#27627=CARTESIAN_POINT('Ctrl Pts',(59.1095633117052,-1.29225919238644,-5.10301614711562));
#27628=CARTESIAN_POINT('Ctrl Pts',(59.6621948906526,1.29225919238629,-5.10301614711619));
#27629=CARTESIAN_POINT('Ctrl Pts',(60.2148264696,3.56527527130572,-3.87292135962584));
#27630=CARTESIAN_POINT('Ctrl Pts',(60.7674580485473,4.97887284148913,-1.70924920544305));
#27631=CARTESIAN_POINT('Ctrl Pts',(61.3200896274947,5.19230067806873,0.866441738717778));
#27632=CARTESIAN_POINT('Ctrl Pts',(61.8727212064421,4.15411146796585,3.23327473773157));
#27633=CARTESIAN_POINT('Ctrl Pts',(62.4253527853894,2.11456331327849,4.82071878586269));
#27634=CARTESIAN_POINT('Ctrl Pts',(62.9779843643369,-0.434705609430122,
5.24611653042845));
#27635=CARTESIAN_POINT('Ctrl Pts',(63.5306159432841,-2.8791876591662,4.40692478284593));
#27636=CARTESIAN_POINT('Ctrl Pts',(64.0832475222316,-4.62963433285796,2.50543280937724));
#27637=CARTESIAN_POINT('Ctrl Pts',(64.6358791011789,-5.26409608723815,3.09085705731855E-10));
#27638=CARTESIAN_POINT('Ctrl Pts',(65.1885106801263,-4.62963433322232,-2.50543281017431));
#27639=CARTESIAN_POINT('Ctrl Pts',(65.7411422590737,-2.87918765822658,-4.40692478140855));
#27640=CARTESIAN_POINT('Ctrl Pts',(66.293773838021,-0.434705611488927,-5.24611653333821));
#27641=CARTESIAN_POINT('Ctrl Pts',(66.8464054169685,2.11456331764827,-4.82071877979622));
#27642=CARTESIAN_POINT('Ctrl Pts',(67.3990369959157,4.15411145875562,-3.23327475046641));
#27643=CARTESIAN_POINT('Ctrl Pts',(67.9516685748631,5.19230069745088,-0.866441711942802));
#27644=CARTESIAN_POINT('Ctrl Pts',(68.5043001538105,4.97887280071541,1.70924914912885));
#27645=CARTESIAN_POINT('Ctrl Pts',(69.0569317327578,3.56527535707346,3.87292147807751));
#27646=CARTESIAN_POINT('Ctrl Pts',(69.6095633117052,1.29225901197643,5.10301589795954));
#27647=CARTESIAN_POINT('Ctrl Pts',(70.1621948906526,-1.29225881290355,5.10301667120488));
#27648=CARTESIAN_POINT('Ctrl Pts',(70.7148264696,-3.56527606954638,3.87292025722596));
#27649=CARTESIAN_POINT('Ctrl Pts',(71.2674580485474,-4.9788711625536,1.70925152427458));
#27650=CARTESIAN_POINT('Ctrl Pts',(71.8200896274948,-5.19230421072891,-0.866446616436202));
#27651=CARTESIAN_POINT('Ctrl Pts',(72.3727212064421,-4.15410404637352,-3.23326447896727));
#27652=CARTESIAN_POINT('Ctrl Pts',(72.9253527853895,-2.11457900308638,-4.82074037636149));
#27653=CARTESIAN_POINT('Ctrl Pts',(73.4779843643368,0.434737962916119,-5.24607120227223));
#27654=CARTESIAN_POINT('Ctrl Pts',(74.0306159432842,2.87911375329489,-4.40702109952745));
#27655=CARTESIAN_POINT('Ctrl Pts',(74.5832475222315,4.62974731329617,-2.50523368528442));
#27656=CARTESIAN_POINT('Ctrl Pts',(74.9516685748631,5.05215470582044,-0.835439667818527));
#27657=CARTESIAN_POINT('Ctrl Pts',(75.1358791011789,5.05215470582044,-7.4245261071363E-15));
#27658=CARTESIAN_POINT('Ctrl Pts',(33.6197755720781,4.94250112032697,0.));
#27659=CARTESIAN_POINT('Ctrl Pts',(33.8039860983939,4.94250112032697,0.817139076837683));
#27660=CARTESIAN_POINT('Ctrl Pts',(34.1724071510254,4.52920068974087,2.45091075495199));
#27661=CARTESIAN_POINT('Ctrl Pts',(34.7250387299729,2.81660319447189,4.31128469373266));
#27662=CARTESIAN_POINT('Ctrl Pts',(35.2776703089202,0.42529402211631,5.13217251323705));
#27663=CARTESIAN_POINT('Ctrl Pts',(35.8303018878676,-2.06865974125642,4.71605075332317));
#27664=CARTESIAN_POINT('Ctrl Pts',(36.3829334668149,-4.06389977762583,3.16305923338873));
#27665=CARTESIAN_POINT('Ctrl Pts',(36.9355650457623,-5.07955447125059,0.847630025952494));
#27666=CARTESIAN_POINT('Ctrl Pts',(37.4881966247097,-4.87075665964084,-1.67213470664358));
#27667=CARTESIAN_POINT('Ctrl Pts',(38.0408282036571,-3.48785707483957,-3.78882139657513));
#27668=CARTESIAN_POINT('Ctrl Pts',(38.5934597826044,-1.26419784346094,-4.9922059811041));
#27669=CARTESIAN_POINT('Ctrl Pts',(39.1460913615518,1.26419801522272,-4.99220553559825));
#27670=CARTESIAN_POINT('Ctrl Pts',(39.6987229404992,3.48785646011191,-3.78882209996813));
#27671=CARTESIAN_POINT('Ctrl Pts',(40.2513545194465,4.87075807306072,-1.67213333819149));
#27672=CARTESIAN_POINT('Ctrl Pts',(40.8039860983939,5.07955143996455,0.847627200316705));
#27673=CARTESIAN_POINT('Ctrl Pts',(41.3566176773413,4.06390617309189,3.16306515207384));
#27674=CARTESIAN_POINT('Ctrl Pts',(41.9092492562886,2.06864620772757,4.71603831708452));
#27675=CARTESIAN_POINT('Ctrl Pts',(42.461880835236,-0.425266109030922,5.13219868216793));
#27676=CARTESIAN_POINT('Ctrl Pts',(43.0145124141834,-2.81666696027288,4.3112297296128));
#27677=CARTESIAN_POINT('Ctrl Pts',(43.5671439931307,-4.52910320957627,2.45102808648086));
#27678=CARTESIAN_POINT('Ctrl Pts',(44.1197755720781,-5.14978781662001,-1.78074231939325E-10));
#27679=CARTESIAN_POINT('Ctrl Pts',(44.6724071510254,-4.5291032092619,-2.45102808602162));
#27680=CARTESIAN_POINT('Ctrl Pts',(45.2250387299728,-2.8166669610836,-4.31122973044095));
#27681=CARTESIAN_POINT('Ctrl Pts',(45.7776703089202,-0.425266107254567,
-5.13219868049148));
#27682=CARTESIAN_POINT('Ctrl Pts',(46.3303018878675,2.06864620395729,-4.71603832057972));
#27683=CARTESIAN_POINT('Ctrl Pts',(46.882933466815,4.06390618103855,-3.16306514473666));
#27684=CARTESIAN_POINT('Ctrl Pts',(47.4355650457623,5.07955142324146,-0.847627215743122));
#27685=CARTESIAN_POINT('Ctrl Pts',(47.9881966247097,4.87075810824064,1.67213337063694));
#27686=CARTESIAN_POINT('Ctrl Pts',(48.540828203657,3.48785638611078,3.78882203172213));
#27687=CARTESIAN_POINT('Ctrl Pts',(49.0934597826044,1.26419817088188,4.99220567914997));
#27688=CARTESIAN_POINT('Ctrl Pts',(49.6460913615518,-1.264198170882,4.99220567914965));
#27689=CARTESIAN_POINT('Ctrl Pts',(50.1987229404991,-3.48785638611033,3.78882203172264));
#27690=CARTESIAN_POINT('Ctrl Pts',(50.7513545194465,-4.87075810824168,1.67213337063594));
#27691=CARTESIAN_POINT('Ctrl Pts',(51.3039860983939,-5.07955142323925,-0.847627215741061));
#27692=CARTESIAN_POINT('Ctrl Pts',(51.8566176773412,-4.06390618104323,-3.16306514474098));
#27693=CARTESIAN_POINT('Ctrl Pts',(52.4092492562886,-2.06864620394743,-4.71603832057063));
#27694=CARTESIAN_POINT('Ctrl Pts',(52.961880835236,0.425266107233821,-5.13219868051061));
#27695=CARTESIAN_POINT('Ctrl Pts',(53.5145124141833,2.81666696112724,-4.31122973040071));
#27696=CARTESIAN_POINT('Ctrl Pts',(54.0671439931307,4.5291032091701,-2.45102808610628));
#27697=CARTESIAN_POINT('Ctrl Pts',(54.6197755720781,5.14978781681311,-5.90029421800548E-15));
#27698=CARTESIAN_POINT('Ctrl Pts',(55.1724071510255,4.52910320917011,2.45102808610628));
#27699=CARTESIAN_POINT('Ctrl Pts',(55.7250387299728,2.81666696112724,4.3112297304007));
#27700=CARTESIAN_POINT('Ctrl Pts',(56.2776703089202,0.425266107233817,5.13219868051062));
#27701=CARTESIAN_POINT('Ctrl Pts',(56.8303018878676,-2.06864620394744,4.71603832057062));
#27702=CARTESIAN_POINT('Ctrl Pts',(57.3829334668149,-4.06390618104323,3.16306514474098));
#27703=CARTESIAN_POINT('Ctrl Pts',(57.9355650457622,-5.07955142323925,0.847627215741054));
#27704=CARTESIAN_POINT('Ctrl Pts',(58.4881966247097,-4.87075810824168,-1.67213337063594));
#27705=CARTESIAN_POINT('Ctrl Pts',(59.0408282036571,-3.48785638611033,-3.78882203172264));
#27706=CARTESIAN_POINT('Ctrl Pts',(59.5934597826044,-1.26419817088201,-4.99220567914965));
#27707=CARTESIAN_POINT('Ctrl Pts',(60.1460913615518,1.26419817088187,-4.99220567914997));
#27708=CARTESIAN_POINT('Ctrl Pts',(60.6987229404992,3.48785638611077,-3.78882203172213));
#27709=CARTESIAN_POINT('Ctrl Pts',(61.2513545194465,4.87075810824064,-1.67213337063695));
#27710=CARTESIAN_POINT('Ctrl Pts',(61.8039860983939,5.07955142324146,0.847627215743118));
#27711=CARTESIAN_POINT('Ctrl Pts',(62.3566176773412,4.06390618103855,3.16306514473665));
#27712=CARTESIAN_POINT('Ctrl Pts',(62.9092492562886,2.06864620395729,4.71603832057972));
#27713=CARTESIAN_POINT('Ctrl Pts',(63.461880835236,-0.425266107254564,5.13219868049148));
#27714=CARTESIAN_POINT('Ctrl Pts',(64.0145124141834,-2.8166669610836,4.31122973044095));
#27715=CARTESIAN_POINT('Ctrl Pts',(64.5671439931307,-4.5291032092619,2.45102808602162));
#27716=CARTESIAN_POINT('Ctrl Pts',(65.1197755720782,-5.14978781662001,1.78081473209479E-10));
#27717=CARTESIAN_POINT('Ctrl Pts',(65.6724071510254,-4.52910320957627,-2.45102808648086));
#27718=CARTESIAN_POINT('Ctrl Pts',(66.2250387299728,-2.81666696027288,-4.3112297296128));
#27719=CARTESIAN_POINT('Ctrl Pts',(66.7776703089202,-0.425266109030917,
-5.13219868216794));
#27720=CARTESIAN_POINT('Ctrl Pts',(67.3303018878675,2.06864620772757,-4.71603831708452));
#27721=CARTESIAN_POINT('Ctrl Pts',(67.8829334668149,4.06390617309189,-3.16306515207384));
#27722=CARTESIAN_POINT('Ctrl Pts',(68.4355650457623,5.07955143996455,-0.847627200316705));
#27723=CARTESIAN_POINT('Ctrl Pts',(68.9881966247097,4.87075807306072,1.67213333819149));
#27724=CARTESIAN_POINT('Ctrl Pts',(69.540828203657,3.48785646011191,3.78882209996812));
#27725=CARTESIAN_POINT('Ctrl Pts',(70.0934597826044,1.26419801522272,4.99220553559826));
#27726=CARTESIAN_POINT('Ctrl Pts',(70.6460913615518,-1.26419784346096,4.99220598110409));
#27727=CARTESIAN_POINT('Ctrl Pts',(71.1987229404992,-3.48785707483957,3.78882139657512));
#27728=CARTESIAN_POINT('Ctrl Pts',(71.7513545194465,-4.87075665964084,1.67213470664358));
#27729=CARTESIAN_POINT('Ctrl Pts',(72.3039860983939,-5.0795544712506,-0.847630025952498));
#27730=CARTESIAN_POINT('Ctrl Pts',(72.8566176773413,-4.06389977762583,-3.16305923338874));
#27731=CARTESIAN_POINT('Ctrl Pts',(73.4092492562886,-2.06865974125642,-4.71605075332316));
#27732=CARTESIAN_POINT('Ctrl Pts',(73.961880835236,0.425294022116303,-5.13217251323706));
#27733=CARTESIAN_POINT('Ctrl Pts',(74.5145124141834,2.81660319447188,-4.31128469373267));
#27734=CARTESIAN_POINT('Ctrl Pts',(75.0671439931307,4.52920068974087,-2.45091075495198));
#27735=CARTESIAN_POINT('Ctrl Pts',(75.4355650457623,4.94250112032697,-0.817139076837684));
#27736=CARTESIAN_POINT('Ctrl Pts',(75.6197755720781,4.94250112032697,-7.26338181214876E-15));
#27737=CARTESIAN_POINT('Ctrl Pts',(33.9441734627902,5.19996900808372,0.));
#27738=CARTESIAN_POINT('Ctrl Pts',(34.128383989106,5.19996900808372,0.859814026526804));
#27739=CARTESIAN_POINT('Ctrl Pts',(34.4968050417376,4.76517797451894,2.57855204094631));
#27740=CARTESIAN_POINT('Ctrl Pts',(35.0494366206849,2.96334119934827,4.53592553639668));
#27741=CARTESIAN_POINT('Ctrl Pts',(35.6020681996323,0.447454012565768,5.39954421798947));
#27742=CARTESIAN_POINT('Ctrl Pts',(36.1546997785797,-2.17643695412734,4.96176002173633));
#27743=CARTESIAN_POINT('Ctrl Pts',(36.707331357527,-4.27562619453865,3.32785024601096));
#27744=CARTESIAN_POINT('Ctrl Pts',(37.2599629364744,-5.34419675899476,0.891792351082074));
#27745=CARTESIAN_POINT('Ctrl Pts',(37.8125945154218,-5.12452030784397,-1.75925261524249));
#27746=CARTESIAN_POINT('Ctrl Pts',(38.3652260943691,-3.66957259079425,-3.98621664555567));
#27747=CARTESIAN_POINT('Ctrl Pts',(38.9178576733165,-1.33006183535942,-5.25229733317933));
#27748=CARTESIAN_POINT('Ctrl Pts',(39.4704892522639,1.33006203085693,-5.25229666444782));
#27749=CARTESIAN_POINT('Ctrl Pts',(40.0231208312112,3.6695718911175,-3.98621770139316));
#27750=CARTESIAN_POINT('Ctrl Pts',(40.5757524101586,5.12452191658404,-1.75925056112342));
#27751=CARTESIAN_POINT('Ctrl Pts',(41.1283839891059,5.34419330881595,0.891788109530082));
#27752=CARTESIAN_POINT('Ctrl Pts',(41.6810155680534,4.27563347379279,3.32785912949593));
#27753=CARTESIAN_POINT('Ctrl Pts',(42.2336471470007,2.17642155040303,4.96174134693238));
#27754=CARTESIAN_POINT('Ctrl Pts',(42.7862787259481,-0.44742224217709,5.39958344300911));
#27755=CARTESIAN_POINT('Ctrl Pts',(43.3389103048954,-2.96341377693166,4.53584245342762));
#27756=CARTESIAN_POINT('Ctrl Pts',(43.8915418838428,-4.76506702359125,2.57872531691644));
#27757=CARTESIAN_POINT('Ctrl Pts',(44.4441734627902,-5.41808896103925,-2.67301766495115E-10));
#27758=CARTESIAN_POINT('Ctrl Pts',(44.9968050417375,-4.76506702323344,-2.5787253162271));
#27759=CARTESIAN_POINT('Ctrl Pts',(45.5494366206849,-2.96341377785441,-4.53584245467072));
#27760=CARTESIAN_POINT('Ctrl Pts',(46.1020681996323,-0.447422240155257,
-5.39958344049266));
#27761=CARTESIAN_POINT('Ctrl Pts',(46.6546997785796,2.17642154611174,-4.96174135217889));
#27762=CARTESIAN_POINT('Ctrl Pts',(47.207331357527,4.27563348283759,-3.32785911848237));
#27763=CARTESIAN_POINT('Ctrl Pts',(47.7599629364744,5.3441932897819,-0.891788132686083));
#27764=CARTESIAN_POINT('Ctrl Pts',(48.3125945154218,5.12452195662546,1.75925060982603));
#27765=CARTESIAN_POINT('Ctrl Pts',(48.8652260943691,3.66957180689017,3.98621759895172));
#27766=CARTESIAN_POINT('Ctrl Pts',(49.4178576733165,1.33006220802659,5.25229687992779));
#27767=CARTESIAN_POINT('Ctrl Pts',(49.9704892522639,-1.33006220802673,5.2522968799273));
#27768=CARTESIAN_POINT('Ctrl Pts',(50.5231208312112,-3.66957180688966,3.9862175989525));
#27769=CARTESIAN_POINT('Ctrl Pts',(51.0757524101586,-5.12452195662665,1.75925060982452));
#27770=CARTESIAN_POINT('Ctrl Pts',(51.628383989106,-5.34419328977938,-0.891788132682984));
#27771=CARTESIAN_POINT('Ctrl Pts',(52.1810155680533,-4.27563348284292,-3.32785911848886));
#27772=CARTESIAN_POINT('Ctrl Pts',(52.7336471470007,-2.17642154610051,-4.96174135216523));
#27773=CARTESIAN_POINT('Ctrl Pts',(53.2862787259481,0.447422240131642,-5.39958344052137));
#27774=CARTESIAN_POINT('Ctrl Pts',(53.8389103048955,2.96341377790408,-4.53584245461031));
#27775=CARTESIAN_POINT('Ctrl Pts',(54.3915418838428,4.76506702312895,-2.57872531635419));
#27776=CARTESIAN_POINT('Ctrl Pts',(54.9441734627902,5.41808896125903,-4.00057827660221E-15));
#27777=CARTESIAN_POINT('Ctrl Pts',(55.4968050417376,4.76506702312896,2.57872531635418));
#27778=CARTESIAN_POINT('Ctrl Pts',(56.0494366206849,2.96341377790408,4.5358424546103));
#27779=CARTESIAN_POINT('Ctrl Pts',(56.6020681996323,0.44742224013164,5.39958344052138));
#27780=CARTESIAN_POINT('Ctrl Pts',(57.1546997785797,-2.17642154610052,4.96174135216522));
#27781=CARTESIAN_POINT('Ctrl Pts',(57.707331357527,-4.27563348284293,3.32785911848886));
#27782=CARTESIAN_POINT('Ctrl Pts',(58.2599629364744,-5.34419328977938,0.89178813268298));
#27783=CARTESIAN_POINT('Ctrl Pts',(58.8125945154218,-5.12452195662665,-1.75925060982453));
#27784=CARTESIAN_POINT('Ctrl Pts',(59.3652260943691,-3.66957180688966,-3.9862175989525));
#27785=CARTESIAN_POINT('Ctrl Pts',(59.9178576733165,-1.33006220802674,-5.2522968799273));
#27786=CARTESIAN_POINT('Ctrl Pts',(60.4704892522639,1.33006220802658,-5.2522968799278));
#27787=CARTESIAN_POINT('Ctrl Pts',(61.0231208312112,3.66957180689017,-3.98621759895173));
#27788=CARTESIAN_POINT('Ctrl Pts',(61.5757524101587,5.12452195662546,-1.75925060982604));
#27789=CARTESIAN_POINT('Ctrl Pts',(62.128383989106,5.3441932897819,0.891788132686079));
#27790=CARTESIAN_POINT('Ctrl Pts',(62.6810155680533,4.27563348283759,3.32785911848237));
#27791=CARTESIAN_POINT('Ctrl Pts',(63.2336471470007,2.17642154611174,4.96174135217889));
#27792=CARTESIAN_POINT('Ctrl Pts',(63.7862787259481,-0.447422240155256,
5.39958344049265));
#27793=CARTESIAN_POINT('Ctrl Pts',(64.3389103048954,-2.96341377785441,4.53584245467072));
#27794=CARTESIAN_POINT('Ctrl Pts',(64.8915418838428,-4.76506702323344,2.57872531622711));
#27795=CARTESIAN_POINT('Ctrl Pts',(65.4441734627902,-5.41808896103925,2.67308784269264E-10));
#27796=CARTESIAN_POINT('Ctrl Pts',(65.9968050417376,-4.76506702359125,-2.57872531691644));
#27797=CARTESIAN_POINT('Ctrl Pts',(66.5494366206849,-2.96341377693166,-4.53584245342762));
#27798=CARTESIAN_POINT('Ctrl Pts',(67.1020681996323,-0.447422242177083,
-5.39958344300911));
#27799=CARTESIAN_POINT('Ctrl Pts',(67.6546997785796,2.17642155040303,-4.96174134693238));
#27800=CARTESIAN_POINT('Ctrl Pts',(68.2073313575271,4.27563347379279,-3.32785912949593));
#27801=CARTESIAN_POINT('Ctrl Pts',(68.7599629364744,5.34419330881595,-0.891788109530083));
#27802=CARTESIAN_POINT('Ctrl Pts',(69.3125945154218,5.12452191658404,1.75925056112342));
#27803=CARTESIAN_POINT('Ctrl Pts',(69.8652260943691,3.6695718911175,3.98621770139316));
#27804=CARTESIAN_POINT('Ctrl Pts',(70.4178576733165,1.33006203085692,5.25229666444782));
#27805=CARTESIAN_POINT('Ctrl Pts',(70.9704892522639,-1.33006183535944,5.25229733317932));
#27806=CARTESIAN_POINT('Ctrl Pts',(71.5231208312112,-3.66957259079425,3.98621664555566));
#27807=CARTESIAN_POINT('Ctrl Pts',(72.0757524101586,-5.12452030784397,1.75925261524249));
#27808=CARTESIAN_POINT('Ctrl Pts',(72.628383989106,-5.34419675899477,-0.891792351082077));
#27809=CARTESIAN_POINT('Ctrl Pts',(73.1810155680534,-4.27562619453864,-3.32785024601098));
#27810=CARTESIAN_POINT('Ctrl Pts',(73.7336471470007,-2.17643695412734,-4.96176002173632));
#27811=CARTESIAN_POINT('Ctrl Pts',(74.2862787259481,0.447454012565758,-5.39954421798947));
#27812=CARTESIAN_POINT('Ctrl Pts',(74.8389103048955,2.96334119934827,-4.53592553639669));
#27813=CARTESIAN_POINT('Ctrl Pts',(75.3915418838428,4.76517797451894,-2.5785520409463));
#27814=CARTESIAN_POINT('Ctrl Pts',(75.7599629364744,5.19996900808372,-0.859814026526805));
#27815=CARTESIAN_POINT('Ctrl Pts',(75.9441734627902,5.19996900808372,-7.6417504816982E-15));
#27816=CARTESIAN_POINT('Ctrl Pts',(33.992328768859,5.42478616651165,0.));
#27817=CARTESIAN_POINT('Ctrl Pts',(34.1765392951748,5.42478616651165,0.897005658049128));
#27818=CARTESIAN_POINT('Ctrl Pts',(34.5449603478064,4.97120383948995,2.69002843971947));
#27819=CARTESIAN_POINT('Ctrl Pts',(35.0975919267537,3.09146156820945,4.73204241007042));
#27820=CARTESIAN_POINT('Ctrl Pts',(35.6502235057011,0.46680027700504,5.63299379713529));
#27821=CARTESIAN_POINT('Ctrl Pts',(36.2028550846485,-2.27053630835485,5.1762847224297));
#27822=CARTESIAN_POINT('Ctrl Pts',(36.7554866635958,-4.46048458163846,3.47173079196878));
#27823=CARTESIAN_POINT('Ctrl Pts',(37.3081182425432,-5.57525537632878,0.930349576908284));
#27824=CARTESIAN_POINT('Ctrl Pts',(37.8607498214906,-5.34608105725119,-1.83531473574165));
#27825=CARTESIAN_POINT('Ctrl Pts',(38.4133814004379,-3.82822810044738,-4.15856233495235));
#27826=CARTESIAN_POINT('Ctrl Pts',(38.9660129793853,-1.3875676081727,-5.47938261924127));
#27827=CARTESIAN_POINT('Ctrl Pts',(39.5186445583327,1.38756781460722,-5.47938188798928));
#27828=CARTESIAN_POINT('Ctrl Pts',(40.07127613728,3.82822736162757,-4.1585634895015));
#27829=CARTESIAN_POINT('Ctrl Pts',(40.6239077162274,5.34608275599143,-1.83531248958194));
#27830=CARTESIAN_POINT('Ctrl Pts',(41.1765392951747,5.57525173313143,0.93034493879696));
#27831=CARTESIAN_POINT('Ctrl Pts',(41.7291708741222,4.46049226812687,3.471740505884));
#27832=CARTESIAN_POINT('Ctrl Pts',(42.2818024530695,2.27052004287681,5.17626430084314));
#27833=CARTESIAN_POINT('Ctrl Pts',(42.8344340320169,-0.466766729237704,
5.6330366827348));
#27834=CARTESIAN_POINT('Ctrl Pts',(43.3870656109642,-3.09153820610978,4.73195149145368));
#27835=CARTESIAN_POINT('Ctrl Pts',(43.9396971899116,-4.97108668146758,2.69021758030695));
#27836=CARTESIAN_POINT('Ctrl Pts',(44.492328768859,-5.65234229441848,-2.92291792167501E-10));
#27837=CARTESIAN_POINT('Ctrl Pts',(45.0449603478063,-4.97108668108975,-2.69021757955316));
#27838=CARTESIAN_POINT('Ctrl Pts',(45.5975919267537,-3.09153820708416,-4.731951492813));
#27839=CARTESIAN_POINT('Ctrl Pts',(46.1502235057011,-0.466766727102762,
-5.63303667998308));
#27840=CARTESIAN_POINT('Ctrl Pts',(46.7028550846484,2.27052003834545,-5.17626430658015));
#27841=CARTESIAN_POINT('Ctrl Pts',(47.2554866635958,4.46049227767768,-3.47174049384076));
#27842=CARTESIAN_POINT('Ctrl Pts',(47.8081182425432,5.57525171303253,-0.930344964117844));
#27843=CARTESIAN_POINT('Ctrl Pts',(48.3607498214906,5.34608279827294,1.83531254283782));
#27844=CARTESIAN_POINT('Ctrl Pts',(48.9133814004379,3.82822727268818,4.15856337748268));
#27845=CARTESIAN_POINT('Ctrl Pts',(49.4660129793853,1.38756800168855,5.47938212361473));
#27846=CARTESIAN_POINT('Ctrl Pts',(50.0186445583327,-1.3875680016887,5.4793821236142));
#27847=CARTESIAN_POINT('Ctrl Pts',(50.57127613728,-3.82822727268764,4.15856337748353));
#27848=CARTESIAN_POINT('Ctrl Pts',(51.1239077162274,-5.34608279827419,1.83531254283617));
#27849=CARTESIAN_POINT('Ctrl Pts',(51.6765392951748,-5.57525171302987,-0.930344964114455));
#27850=CARTESIAN_POINT('Ctrl Pts',(52.2291708741221,-4.46049227768331,-3.47174049384787));
#27851=CARTESIAN_POINT('Ctrl Pts',(52.7818024530695,-2.27052003833359,-5.17626430656522));
#27852=CARTESIAN_POINT('Ctrl Pts',(53.3344340320169,0.466766727077827,-5.63303668001448));
#27853=CARTESIAN_POINT('Ctrl Pts',(53.8870656109643,3.09153820713661,-4.73195149274695));
#27854=CARTESIAN_POINT('Ctrl Pts',(54.4396971899116,4.97108668097941,-2.69021757969212));
#27855=CARTESIAN_POINT('Ctrl Pts',(54.992328768859,5.65234229465055,-4.82192605126774E-15));
#27856=CARTESIAN_POINT('Ctrl Pts',(55.5449603478064,4.97108668097942,2.69021757969212));
#27857=CARTESIAN_POINT('Ctrl Pts',(56.0975919267537,3.09153820713661,4.73195149274694));
#27858=CARTESIAN_POINT('Ctrl Pts',(56.6502235057011,0.466766727077823,5.63303668001448));
#27859=CARTESIAN_POINT('Ctrl Pts',(57.2028550846485,-2.2705200383336,5.17626430656521));
#27860=CARTESIAN_POINT('Ctrl Pts',(57.7554866635958,-4.46049227768332,3.47174049384786));
#27861=CARTESIAN_POINT('Ctrl Pts',(58.3081182425432,-5.57525171302987,0.930344964114451));
#27862=CARTESIAN_POINT('Ctrl Pts',(58.8607498214906,-5.34608279827419,-1.83531254283618));
#27863=CARTESIAN_POINT('Ctrl Pts',(59.4133814004379,-3.82822727268764,-4.15856337748353));
#27864=CARTESIAN_POINT('Ctrl Pts',(59.9660129793853,-1.3875680016887,-5.47938212361419));
#27865=CARTESIAN_POINT('Ctrl Pts',(60.5186445583327,1.38756800168854,-5.47938212361474));
#27866=CARTESIAN_POINT('Ctrl Pts',(61.07127613728,3.82822727268818,-4.15856337748269));
#27867=CARTESIAN_POINT('Ctrl Pts',(61.6239077162275,5.34608279827295,-1.83531254283783));
#27868=CARTESIAN_POINT('Ctrl Pts',(62.1765392951748,5.57525171303254,0.93034496411784));
#27869=CARTESIAN_POINT('Ctrl Pts',(62.7291708741221,4.46049227767768,3.47174049384076));
#27870=CARTESIAN_POINT('Ctrl Pts',(63.2818024530695,2.27052003834545,5.17626430658015));
#27871=CARTESIAN_POINT('Ctrl Pts',(63.8344340320169,-0.466766727102761,
5.63303667998307));
#27872=CARTESIAN_POINT('Ctrl Pts',(64.3870656109642,-3.09153820708416,4.731951492813));
#27873=CARTESIAN_POINT('Ctrl Pts',(64.9396971899116,-4.97108668108975,2.69021757955317));
#27874=CARTESIAN_POINT('Ctrl Pts',(65.492328768859,-5.65234229441848,2.92299128423437E-10));
#27875=CARTESIAN_POINT('Ctrl Pts',(66.0449603478064,-4.97108668146758,-2.69021758030695));
#27876=CARTESIAN_POINT('Ctrl Pts',(66.5975919267537,-3.09153820610978,-4.73195149145368));
#27877=CARTESIAN_POINT('Ctrl Pts',(67.1502235057011,-0.466766729237698,
-5.6330366827348));
#27878=CARTESIAN_POINT('Ctrl Pts',(67.7028550846484,2.27052004287681,-5.17626430084314));
#27879=CARTESIAN_POINT('Ctrl Pts',(68.2554866635959,4.46049226812687,-3.471740505884));
#27880=CARTESIAN_POINT('Ctrl Pts',(68.8081182425432,5.57525173313144,-0.930344938796962));
#27881=CARTESIAN_POINT('Ctrl Pts',(69.3607498214906,5.34608275599143,1.83531248958194));
#27882=CARTESIAN_POINT('Ctrl Pts',(69.9133814004379,3.82822736162757,4.15856348950149));
#27883=CARTESIAN_POINT('Ctrl Pts',(70.4660129793853,1.38756781460721,5.47938188798929));
#27884=CARTESIAN_POINT('Ctrl Pts',(71.0186445583327,-1.38756760817271,5.47938261924127));
#27885=CARTESIAN_POINT('Ctrl Pts',(71.5712761372801,-3.82822810044738,4.15856233495234));
#27886=CARTESIAN_POINT('Ctrl Pts',(72.1239077162274,-5.34608105725119,1.83531473574165));
#27887=CARTESIAN_POINT('Ctrl Pts',(72.6765392951748,-5.57525537632879,-0.930349576908287));
#27888=CARTESIAN_POINT('Ctrl Pts',(73.2291708741222,-4.46048458163846,-3.4717307919688));
#27889=CARTESIAN_POINT('Ctrl Pts',(73.7818024530695,-2.27053630835485,-5.1762847224297));
#27890=CARTESIAN_POINT('Ctrl Pts',(74.3344340320169,0.46680027700503,-5.63299379713529));
#27891=CARTESIAN_POINT('Ctrl Pts',(74.8870656109643,3.09146156820945,-4.73204241007043));
#27892=CARTESIAN_POINT('Ctrl Pts',(75.4396971899116,4.97120383948995,-2.69002843971946));
#27893=CARTESIAN_POINT('Ctrl Pts',(75.8081182425432,5.42478616651165,-0.897005658049129));
#27894=CARTESIAN_POINT('Ctrl Pts',(75.992328768859,5.42478616651165,-7.9721364178528E-15));
#27895=CARTESIAN_POINT('Ctrl Pts',(33.9921997677122,5.49976642738082,0.));
#27896=CARTESIAN_POINT('Ctrl Pts',(34.176410294028,5.49976642738082,0.909403588662882));
#27897=CARTESIAN_POINT('Ctrl Pts',(34.5448313466596,5.03991467318512,2.72720954086847));
#27898=CARTESIAN_POINT('Ctrl Pts',(35.0974629256069,3.13419106663809,4.79744756259311));
#27899=CARTESIAN_POINT('Ctrl Pts',(35.6500945045543,0.473252278446431,5.71085179682633));
#27900=CARTESIAN_POINT('Ctrl Pts',(36.2027260835017,-2.30191914515453,5.24783014539696));
#27901=CARTESIAN_POINT('Ctrl Pts',(36.755357662449,-4.52213639346893,3.51971627798693));
#27902=CARTESIAN_POINT('Ctrl Pts',(37.3079892413964,-5.6523152960574,0.943208655172099));
#27903=CARTESIAN_POINT('Ctrl Pts',(37.8606208203438,-5.41997338236277,-1.86068203981508));
#27904=CARTESIAN_POINT('Ctrl Pts',(38.4132523992911,-3.88114100434969,-4.2160410449643));
#27905=CARTESIAN_POINT('Ctrl Pts',(38.9658839782385,-1.40674625429844,-5.55511740772306));
#27906=CARTESIAN_POINT('Ctrl Pts',(39.5185155571859,1.40674646354598,-5.55511666690852));
#27907=CARTESIAN_POINT('Ctrl Pts',(40.0711471361332,3.88114025546219,-4.21604221461142));
#27908=CARTESIAN_POINT('Ctrl Pts',(40.6237787150806,5.41997510425126,-1.86067976428242));
#27909=CARTESIAN_POINT('Ctrl Pts',(41.1764102940279,5.65231160321522,0.943203956408585));
#27910=CARTESIAN_POINT('Ctrl Pts',(41.7290418729754,4.52214418469897,3.51972611893208));
#27911=CARTESIAN_POINT('Ctrl Pts',(42.2816734519227,2.30190265803137,5.24780945677143));
#27912=CARTESIAN_POINT('Ctrl Pts',(42.8343050308701,-0.473218273533045,
5.71089524334113));
#27913=CARTESIAN_POINT('Ctrl Pts',(43.3869366098174,-3.13426874886167,4.79735545609104));
#27914=CARTESIAN_POINT('Ctrl Pts',(43.9395681887648,-5.03979591868312,2.72740116002078));
#27915=CARTESIAN_POINT('Ctrl Pts',(44.4921997677122,-5.73046769283071,-2.96113953592807E-10));
#27916=CARTESIAN_POINT('Ctrl Pts',(45.0448313466595,-5.03979591830015,-2.72740115925713));
#27917=CARTESIAN_POINT('Ctrl Pts',(45.5974629256069,-3.13426874984933,-4.79735545746814));
#27918=CARTESIAN_POINT('Ctrl Pts',(46.1500945045543,-0.473218271369011,
-5.71089524055342));
#27919=CARTESIAN_POINT('Ctrl Pts',(46.7027260835016,2.30190265343826,-5.24780946258346));
#27920=CARTESIAN_POINT('Ctrl Pts',(47.255357662449,4.52214419437993,-3.51972610673135));
#27921=CARTESIAN_POINT('Ctrl Pts',(47.8079892413964,5.65231158284243,-0.943203982060589));
#27922=CARTESIAN_POINT('Ctrl Pts',(48.3606208203438,5.41997514710894,1.86067981823473));
#27923=CARTESIAN_POINT('Ctrl Pts',(48.9132523992911,3.88114016531086,4.21604210112774));
#27924=CARTESIAN_POINT('Ctrl Pts',(49.4658839782385,1.40674665317661,5.55511690561523));
#27925=CARTESIAN_POINT('Ctrl Pts',(50.0185155571858,-1.40674665317677,5.5551169056147));
#27926=CARTESIAN_POINT('Ctrl Pts',(50.5711471361332,-3.8811401653103,4.2160421011286));
#27927=CARTESIAN_POINT('Ctrl Pts',(51.1237787150806,-5.4199751471102,1.86067981823306));
#27928=CARTESIAN_POINT('Ctrl Pts',(51.676410294028,-5.65231158283973,-0.943203982057156));
#27929=CARTESIAN_POINT('Ctrl Pts',(52.2290418729753,-4.52214419438563,-3.51972610673855));
#27930=CARTESIAN_POINT('Ctrl Pts',(52.7816734519227,-2.30190265342625,-5.24780946256834));
#27931=CARTESIAN_POINT('Ctrl Pts',(53.3343050308701,0.473218271343736,-5.71089524058523));
#27932=CARTESIAN_POINT('Ctrl Pts',(53.8869366098175,3.13426874990249,-4.79735545740122));
#27933=CARTESIAN_POINT('Ctrl Pts',(54.4395681887648,5.0397959181883,-2.72740115939791));
#27934=CARTESIAN_POINT('Ctrl Pts',(54.9921997677122,5.73046769306595,-5.11805824213355E-15));
#27935=CARTESIAN_POINT('Ctrl Pts',(55.5448313466596,5.03979591818831,2.72740115939791));
#27936=CARTESIAN_POINT('Ctrl Pts',(56.0974629256069,3.13426874990249,4.79735545740121));
#27937=CARTESIAN_POINT('Ctrl Pts',(56.6500945045543,0.473218271343732,5.71089524058523));
#27938=CARTESIAN_POINT('Ctrl Pts',(57.2027260835016,-2.30190265342626,5.24780946256833));
#27939=CARTESIAN_POINT('Ctrl Pts',(57.755357662449,-4.52214419438564,3.51972610673854));
#27940=CARTESIAN_POINT('Ctrl Pts',(58.3079892413963,-5.65231158283973,0.943203982057152));
#27941=CARTESIAN_POINT('Ctrl Pts',(58.8606208203438,-5.4199751471102,-1.86067981823306));
#27942=CARTESIAN_POINT('Ctrl Pts',(59.4132523992911,-3.88114016531031,-4.2160421011286));
#27943=CARTESIAN_POINT('Ctrl Pts',(59.9658839782385,-1.40674665317677,-5.55511690561469));
#27944=CARTESIAN_POINT('Ctrl Pts',(60.5185155571859,1.40674665317661,-5.55511690561524));
#27945=CARTESIAN_POINT('Ctrl Pts',(61.0711471361332,3.88114016531085,-4.21604210112775));
#27946=CARTESIAN_POINT('Ctrl Pts',(61.6237787150807,5.41997514710894,-1.86067981823474));
#27947=CARTESIAN_POINT('Ctrl Pts',(62.1764102940279,5.65231158284244,0.943203982060585));
#27948=CARTESIAN_POINT('Ctrl Pts',(62.7290418729753,4.52214419437993,3.51972610673135));
#27949=CARTESIAN_POINT('Ctrl Pts',(63.2816734519227,2.30190265343826,5.24780946258346));
#27950=CARTESIAN_POINT('Ctrl Pts',(63.8343050308701,-0.473218271369009,
5.71089524055341));
#27951=CARTESIAN_POINT('Ctrl Pts',(64.3869366098174,-3.13426874984932,4.79735545746814));
#27952=CARTESIAN_POINT('Ctrl Pts',(64.9395681887648,-5.03979591830014,2.72740115925714));
#27953=CARTESIAN_POINT('Ctrl Pts',(65.4921997677122,-5.73046769283071,2.96121409977839E-10));
#27954=CARTESIAN_POINT('Ctrl Pts',(66.0448313466595,-5.03979591868312,-2.72740116002078));
#27955=CARTESIAN_POINT('Ctrl Pts',(66.5974629256069,-3.13426874886167,-4.79735545609105));
#27956=CARTESIAN_POINT('Ctrl Pts',(67.1500945045543,-0.473218273533038,
-5.71089524334112));
#27957=CARTESIAN_POINT('Ctrl Pts',(67.7027260835016,2.30190265803138,-5.24780945677143));
#27958=CARTESIAN_POINT('Ctrl Pts',(68.255357662449,4.52214418469897,-3.51972611893208));
#27959=CARTESIAN_POINT('Ctrl Pts',(68.8079892413964,5.65231160321522,-0.943203956408587));
#27960=CARTESIAN_POINT('Ctrl Pts',(69.3606208203438,5.41997510425126,1.86067976428242));
#27961=CARTESIAN_POINT('Ctrl Pts',(69.9132523992911,3.88114025546219,4.21604221461142));
#27962=CARTESIAN_POINT('Ctrl Pts',(70.4658839782385,1.40674646354597,5.55511666690853));
#27963=CARTESIAN_POINT('Ctrl Pts',(71.0185155571859,-1.40674625429845,5.55511740772306));
#27964=CARTESIAN_POINT('Ctrl Pts',(71.5711471361332,-3.8811410043497,4.21604104496428));
#27965=CARTESIAN_POINT('Ctrl Pts',(72.1237787150806,-5.41997338236277,1.86068203981508));
#27966=CARTESIAN_POINT('Ctrl Pts',(72.676410294028,-5.65231529605741,-0.943208655172103));
#27967=CARTESIAN_POINT('Ctrl Pts',(73.2290418729754,-4.52213639346892,-3.51971627798694));
#27968=CARTESIAN_POINT('Ctrl Pts',(73.7816734519227,-2.30191914515453,-5.24783014539695));
#27969=CARTESIAN_POINT('Ctrl Pts',(74.3343050308701,0.473252278446422,-5.71085179682633));
#27970=CARTESIAN_POINT('Ctrl Pts',(74.8869366098175,3.13419106663809,-4.79744756259312));
#27971=CARTESIAN_POINT('Ctrl Pts',(75.4395681887648,5.03991467318512,-2.72720954086847));
#27972=CARTESIAN_POINT('Ctrl Pts',(75.8079892413964,5.49976642738082,-0.909403588662883));
#27973=CARTESIAN_POINT('Ctrl Pts',(75.9921997677122,5.49976642738082,-8.08232562162E-15));
#27974=CARTESIAN_POINT('Ctrl Pts',(33.9921997677122,5.49976642738082,5.17361254957654E-35));
#27975=CARTESIAN_POINT('Ctrl Pts',(33.9921996337599,5.49984428540435,5.17361254957654E-35));
#27976=CARTESIAN_POINT('Ctrl Pts',(33.9921994823618,5.49992214302643,0.));
#27977=CARTESIAN_POINT('Ctrl Pts',(33.9921993135185,5.50000000023809,0.));
#27978=CARTESIAN_POINT('Ctrl Pts',(33.9921134030113,5.53961514866854,0.));
#27979=CARTESIAN_POINT('Ctrl Pts',(33.9875106886727,5.57927270787206,0.));
#27980=CARTESIAN_POINT('Ctrl Pts',(33.9693064765724,5.65615401280177,0.));
#27981=CARTESIAN_POINT('Ctrl Pts',(33.955725697793,5.69351111459438,0.));
#27982=CARTESIAN_POINT('Ctrl Pts',(33.9070143140728,5.78787293252881,0.));
#27983=CARTESIAN_POINT('Ctrl Pts',(33.8641799465949,5.84036554141816,0.));
#27984=CARTESIAN_POINT('Ctrl Pts',(33.7655175445174,5.92324377184529,0.));
#27985=CARTESIAN_POINT('Ctrl Pts',(33.7103194075936,5.9548999521189,0.));
#27986=CARTESIAN_POINT('Ctrl Pts',(33.5834982245157,5.99813254826451,0.));
#27987=CARTESIAN_POINT('Ctrl Pts',(33.5193764033541,6.00295356243643,0.));
#27988=CARTESIAN_POINT('Ctrl Pts',(33.3972845623173,5.99470928422369,0.));
#27989=CARTESIAN_POINT('Ctrl Pts',(33.3323414527145,5.97758452130161,0.));
#27990=CARTESIAN_POINT('Ctrl Pts',(33.2112723468849,5.91926289378582,0.));
#27991=CARTESIAN_POINT('Ctrl Pts',(33.1613177334755,5.8799704596013,0.));
#27992=CARTESIAN_POINT('Ctrl Pts',(33.0761471586416,5.78359940593522,0.));
#27993=CARTESIAN_POINT('Ctrl Pts',(33.0420370989278,5.72456593715523,0.));
#27994=CARTESIAN_POINT('Ctrl Pts',(33.0050967455162,5.6177642498931,0.));
#27995=CARTESIAN_POINT('Ctrl Pts',(32.9926516271063,5.56306095689167,-1.33481475863792E-22));
#27996=CARTESIAN_POINT('Ctrl Pts',(32.9926516271063,5.5,-1.33481475863792E-22));
#27997=CARTESIAN_POINT('Ctrl Pts',(75.9921997677122,5.49976642738082,-8.88178419700125E-15));
#27998=CARTESIAN_POINT('Ctrl Pts',(75.99219963376,5.49984428532499,-8.88189861517979E-15));
#27999=CARTESIAN_POINT('Ctrl Pts',(75.9921994823621,5.4999221428677,-8.88203003829887E-15));
#28000=CARTESIAN_POINT('Ctrl Pts',(75.992199313519,5.5,-8.88214445528432E-15));
#28001=CARTESIAN_POINT('Ctrl Pts',(75.9921134030299,5.53961514843935,-8.94036193296511E-15));
#28002=CARTESIAN_POINT('Ctrl Pts',(75.9875106887073,5.57927270765391,-9.00722814171805E-15));
#28003=CARTESIAN_POINT('Ctrl Pts',(75.9693064766338,5.65615401261384,-9.1202110745582E-15));
#28004=CARTESIAN_POINT('Ctrl Pts',(75.955725697865,5.69351111442127,-8.84808572513712E-15));
#28005=CARTESIAN_POINT('Ctrl Pts',(75.9070143141801,5.78787293237739,-8.98675760312315E-15));
#28006=CARTESIAN_POINT('Ctrl Pts',(75.8641799467243,5.84036554127547,-9.07499142441514E-15));
#28007=CARTESIAN_POINT('Ctrl Pts',(75.7655175446779,5.92324377174254,-9.19678729600774E-15));
#28008=CARTESIAN_POINT('Ctrl Pts',(75.7103194077563,5.95489995203899,-9.24849061649267E-15));
#28009=CARTESIAN_POINT('Ctrl Pts',(75.583498224688,5.99813254823382,-9.31202420915126E-15));
#28010=CARTESIAN_POINT('Ctrl Pts',(75.5193764035373,6.00295356242793,-9.45958558899066E-15));
#28011=CARTESIAN_POINT('Ctrl Pts',(75.3972845624903,5.99470928425966,-9.4474699943466E-15));
#28012=CARTESIAN_POINT('Ctrl Pts',(75.3323414528765,5.9775845213551,-9.4182367933636E-15));
#28013=CARTESIAN_POINT('Ctrl Pts',(75.2112723471179,5.91926289392378,-9.3325287201378E-15));
#28014=CARTESIAN_POINT('Ctrl Pts',(75.1613177336804,5.879970459797,-9.41550176458032E-15));
#28015=CARTESIAN_POINT('Ctrl Pts',(75.0761471587424,5.78359940608845,-9.27387716163476E-15));
#28016=CARTESIAN_POINT('Ctrl Pts',(75.0420370990085,5.72456593731634,-9.17263343837334E-15));
#28017=CARTESIAN_POINT('Ctrl Pts',(75.005096745547,5.61776425003271,-9.01568022500282E-15));
#28018=CARTESIAN_POINT('Ctrl Pts',(74.9926516271063,5.56306095696798,-8.97445707592366E-15));
#28019=CARTESIAN_POINT('Ctrl Pts',(74.9926516271063,5.5,-8.88178419700125E-15));
#28020=CARTESIAN_POINT('Origin',(75.4926516271063,5.5,-8.08266887437253E-15));
#28021=CARTESIAN_POINT('Origin',(33.4926516271063,5.5,0.));
#28042=UNCERTAINTY_MEASURE_WITH_UNIT(LENGTH_MEASURE(0.01),#28056,
'DISTANCE_ACCURACY_VALUE',
'Maximum model space distance between geometric entities at asserted c
onnectivities');
#28043=UNCERTAINTY_MEASURE_WITH_UNIT(LENGTH_MEASURE(0.01),#28056,
'DISTANCE_ACCURACY_VALUE',
'Maximum model space distance between geometric entities at asserted c
onnectivities');
#28054=(
GEOMETRIC_REPRESENTATION_CONTEXT(3)
GLOBAL_UNCERTAINTY_ASSIGNED_CONTEXT((#28042))
GLOBAL_UNIT_ASSIGNED_CONTEXT((#28056,#28058,#28059))
REPRESENTATION_CONTEXT('','3D')
);
#28055=(
GEOMETRIC_REPRESENTATION_CONTEXT(3)
GLOBAL_UNCERTAINTY_ASSIGNED_CONTEXT((#28043))
GLOBAL_UNIT_ASSIGNED_CONTEXT((#28056,#28058,#28059))
REPRESENTATION_CONTEXT('','3D')
);
#28056=(
LENGTH_UNIT()
NAMED_UNIT(*)
SI_UNIT(.MILLI.,.METRE.)
);
#28058=(
NAMED_UNIT(*)
PLANE_ANGLE_UNIT()
SI_UNIT($,.RADIAN.)
);
#28059=(
NAMED_UNIT(*)
SI_UNIT($,.STERADIAN.)
SOLID_ANGLE_UNIT()
);
#28070=SHAPE_DEFINITION_REPRESENTATION(#28081,#28102);
#28081=PRODUCT_DEFINITION_SHAPE('',$,#28114);
#28102=SHAPE_REPRESENTATION('',(#4101),#28054);
#28103=PRODUCT_DEFINITION_CONTEXT('part definition',#28138,'design');
#28114=PRODUCT_DEFINITION('Spring','Spring',#28125,#28103);
#28125=PRODUCT_DEFINITION_FORMATION('',$,#28150);
#28138=APPLICATION_CONTEXT(
'Core Data for Automotive Mechanical Design Process');
#28139=PRODUCT_CONTEXT('part definition',#28138,'mechanical');
#28150=PRODUCT('Spring','Spring',$,(#28139));
#28152=PRESENTATION_STYLE_ASSIGNMENT((#28155));
#28155=SURFACE_STYLE_USAGE(.BOTH.,#28158);
#28158=SURFACE_SIDE_STYLE('',(#28161));
#28161=SURFACE_STYLE_FILL_AREA(#28164);
#28164=FILL_AREA_STYLE('Opaque(160,160,160)',(#28167));
#28167=FILL_AREA_STYLE_COLOUR('Opaque(160,160,160)',#28170);
#28170=COLOUR_RGB('Opaque(160,160,160)', 0.66274510, 0.83137255, 0.94901961);
ENDSEC;
END-ISO-10303-21;
